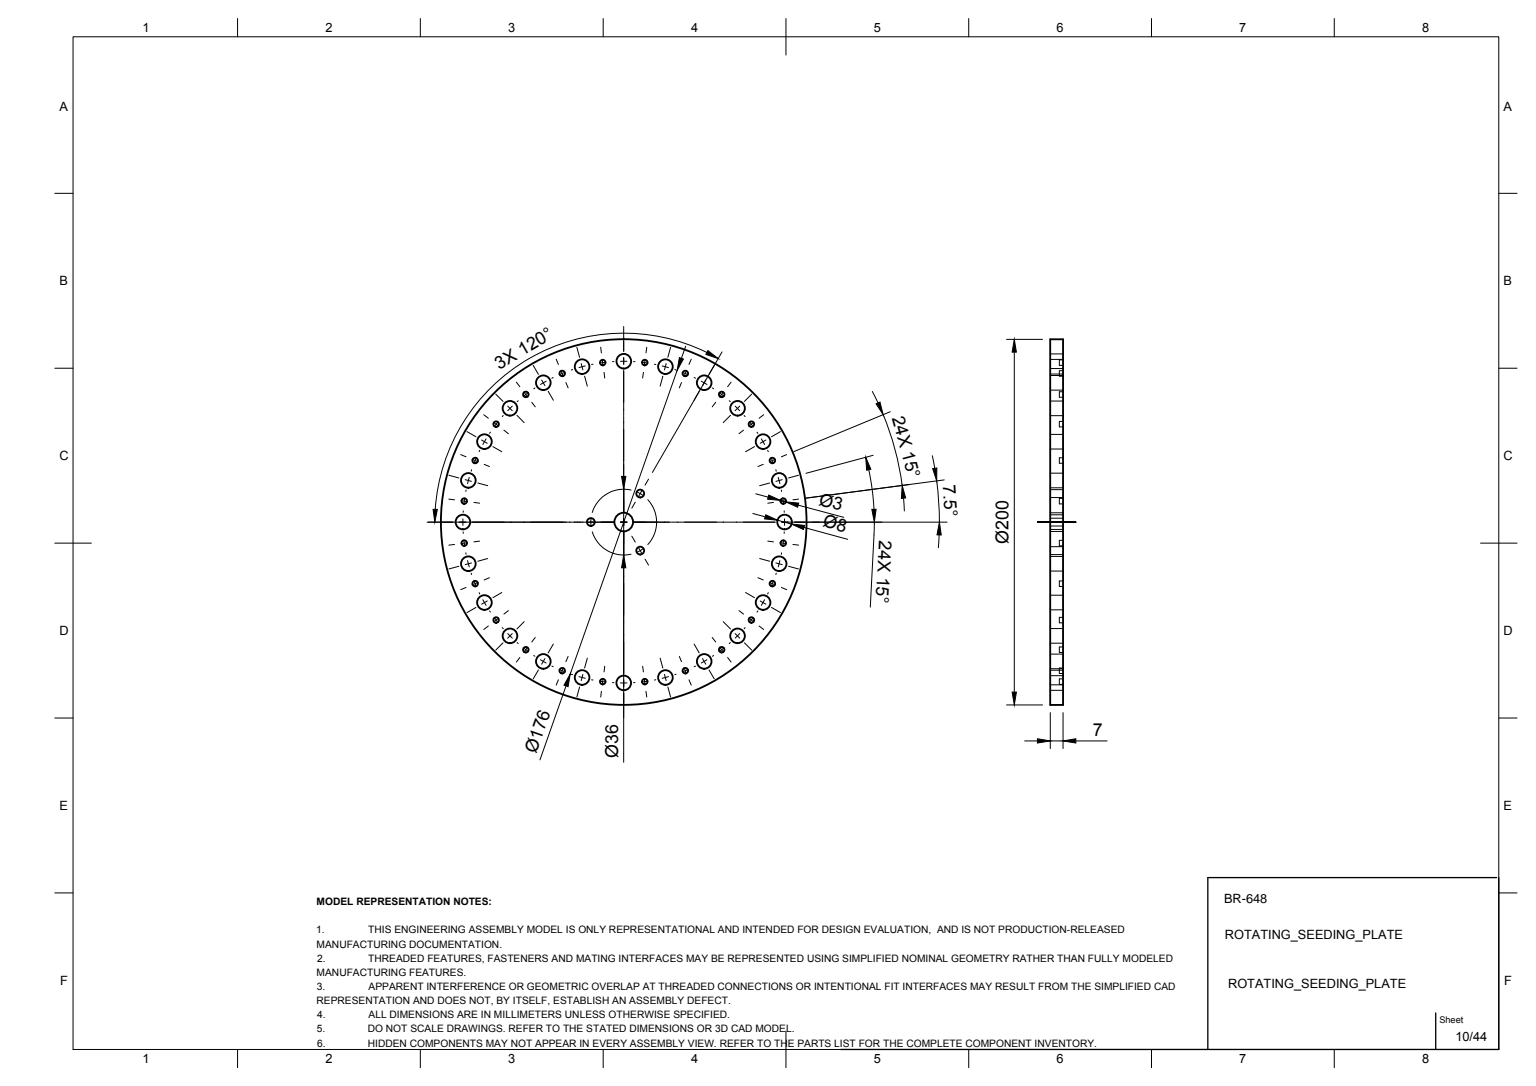
ISO-10303-21;
HEADER;
FILE_DESCRIPTION((''),'2;1');
FILE_NAME('ROTATING_SEEDING_PLATE.step','2026-10-01T22:05:39-07:00',(''),(''),'','','');
FILE_SCHEMA (('AUTOMOTIVE_DESIGN { 1 0 10303 214 3 1 1 }'));
ENDSEC;
DATA;
#10=MECHANICAL_DESIGN_GEOMETRIC_PRESENTATION_REPRESENTATION('',(#610),#24628);
#526=SHAPE_REPRESENTATION_RELATIONSHIP('SRR','None',#24798,#568) ;
#568=ADVANCED_BREP_SHAPE_REPRESENTATION('',(#652),#24588) ;
#610=STYLED_ITEM('',(#25034),#652) ;
#652=MANIFOLD_SOLID_BREP('ROTATING_SEEDING_PLATE',#13119) ;
#759=FACE_BOUND('',#3963,.T.) ;
#760=FACE_BOUND('',#3964,.T.) ;
#761=FACE_BOUND('',#3965,.T.) ;
#762=FACE_BOUND('',#3966,.T.) ;
#763=FACE_BOUND('',#3967,.T.) ;
#764=FACE_BOUND('',#3968,.T.) ;
#765=FACE_BOUND('',#3969,.T.) ;
#766=FACE_BOUND('',#3970,.T.) ;
#767=FACE_BOUND('',#3971,.T.) ;
#768=FACE_BOUND('',#3972,.T.) ;
#769=FACE_BOUND('',#3973,.T.) ;
#770=FACE_BOUND('',#3974,.T.) ;
#771=FACE_BOUND('',#3975,.T.) ;
#772=FACE_BOUND('',#3976,.T.) ;
#773=FACE_BOUND('',#3977,.T.) ;
#774=FACE_BOUND('',#3978,.T.) ;
#775=FACE_BOUND('',#3979,.T.) ;
#776=FACE_BOUND('',#3980,.T.) ;
#777=FACE_BOUND('',#3981,.T.) ;
#778=FACE_BOUND('',#3982,.T.) ;
#779=FACE_BOUND('',#3983,.T.) ;
#780=FACE_BOUND('',#3984,.T.) ;
#781=FACE_BOUND('',#3985,.T.) ;
#782=FACE_BOUND('',#3986,.T.) ;
#783=FACE_BOUND('',#3987,.T.) ;
#784=FACE_BOUND('',#3988,.T.) ;
#785=FACE_BOUND('',#3989,.T.) ;
#786=FACE_BOUND('',#3990,.T.) ;
#787=FACE_BOUND('',#3991,.T.) ;
#788=FACE_BOUND('',#3992,.T.) ;
#789=FACE_BOUND('',#3993,.T.) ;
#790=FACE_BOUND('',#3994,.T.) ;
#791=FACE_BOUND('',#3995,.T.) ;
#792=FACE_BOUND('',#3996,.T.) ;
#793=FACE_BOUND('',#3997,.T.) ;
#794=FACE_BOUND('',#3998,.T.) ;
#795=FACE_BOUND('',#3999,.T.) ;
#796=FACE_BOUND('',#4000,.T.) ;
#797=FACE_BOUND('',#4001,.T.) ;
#798=FACE_BOUND('',#4002,.T.) ;
#799=FACE_BOUND('',#4003,.T.) ;
#800=FACE_BOUND('',#4004,.T.) ;
#801=FACE_BOUND('',#4005,.T.) ;
#802=FACE_BOUND('',#4006,.T.) ;
#803=FACE_BOUND('',#4007,.T.) ;
#804=FACE_BOUND('',#4008,.T.) ;
#805=FACE_BOUND('',#4009,.T.) ;
#806=FACE_BOUND('',#4010,.T.) ;
#807=FACE_BOUND('',#4011,.T.) ;
#808=FACE_BOUND('',#4012,.T.) ;
#809=FACE_BOUND('',#4013,.T.) ;
#810=FACE_BOUND('',#4014,.T.) ;
#811=FACE_BOUND('',#4016,.T.) ;
#812=FACE_BOUND('',#4017,.T.) ;
#813=FACE_BOUND('',#4018,.T.) ;
#814=FACE_BOUND('',#4019,.T.) ;
#815=FACE_BOUND('',#4020,.T.) ;
#816=FACE_BOUND('',#4021,.T.) ;
#817=FACE_BOUND('',#4022,.T.) ;
#818=FACE_BOUND('',#4023,.T.) ;
#819=FACE_BOUND('',#4024,.T.) ;
#820=FACE_BOUND('',#4025,.T.) ;
#821=FACE_BOUND('',#4026,.T.) ;
#822=FACE_BOUND('',#4027,.T.) ;
#823=FACE_BOUND('',#4028,.T.) ;
#824=FACE_BOUND('',#4029,.T.) ;
#825=FACE_BOUND('',#4030,.T.) ;
#826=FACE_BOUND('',#4031,.T.) ;
#827=FACE_BOUND('',#4032,.T.) ;
#828=FACE_BOUND('',#4033,.T.) ;
#829=FACE_BOUND('',#4034,.T.) ;
#830=FACE_BOUND('',#4035,.T.) ;
#831=FACE_BOUND('',#4036,.T.) ;
#832=FACE_BOUND('',#4037,.T.) ;
#833=FACE_BOUND('',#4038,.T.) ;
#834=FACE_BOUND('',#4039,.T.) ;
#835=FACE_BOUND('',#4040,.T.) ;
#836=FACE_BOUND('',#4041,.T.) ;
#837=FACE_BOUND('',#4042,.T.) ;
#838=FACE_BOUND('',#4043,.T.) ;
#1089=LINE('',#20269,#1925) ;
#1090=LINE('',#20276,#1926) ;
#1091=LINE('',#20283,#1927) ;
#1092=LINE('',#20290,#1928) ;
#1093=LINE('',#20297,#1929) ;
#1094=LINE('',#20304,#1930) ;
#1095=LINE('',#20311,#1931) ;
#1096=LINE('',#20318,#1932) ;
#1097=LINE('',#20325,#1933) ;
#1098=LINE('',#20332,#1934) ;
#1099=LINE('',#20339,#1935) ;
#1100=LINE('',#20346,#1936) ;
#1101=LINE('',#20353,#1937) ;
#1102=LINE('',#20360,#1938) ;
#1103=LINE('',#20367,#1939) ;
#1104=LINE('',#20374,#1940) ;
#1105=LINE('',#20381,#1941) ;
#1106=LINE('',#20388,#1942) ;
#1107=LINE('',#20395,#1943) ;
#1108=LINE('',#20402,#1944) ;
#1109=LINE('',#20409,#1945) ;
#1110=LINE('',#20416,#1946) ;
#1111=LINE('',#20423,#1947) ;
#1112=LINE('',#20430,#1948) ;
#1113=LINE('',#20437,#1949) ;
#1114=LINE('',#20443,#1950) ;
#1115=LINE('',#20449,#1951) ;
#1116=LINE('',#20455,#1952) ;
#1117=LINE('',#20461,#1953) ;
#1118=LINE('',#20467,#1954) ;
#1119=LINE('',#20473,#1955) ;
#1120=LINE('',#20479,#1956) ;
#1121=LINE('',#20485,#1957) ;
#1122=LINE('',#20491,#1958) ;
#1123=LINE('',#20497,#1959) ;
#1124=LINE('',#20503,#1960) ;
#1125=LINE('',#20509,#1961) ;
#1126=LINE('',#20515,#1962) ;
#1127=LINE('',#20521,#1963) ;
#1128=LINE('',#20527,#1964) ;
#1129=LINE('',#20533,#1965) ;
#1130=LINE('',#20539,#1966) ;
#1131=LINE('',#20545,#1967) ;
#1132=LINE('',#20551,#1968) ;
#1133=LINE('',#20557,#1969) ;
#1134=LINE('',#20563,#1970) ;
#1135=LINE('',#20569,#1971) ;
#1136=LINE('',#20575,#1972) ;
#1137=LINE('',#20581,#1973) ;
#1138=LINE('',#20587,#1974) ;
#1139=LINE('',#20593,#1975) ;
#1140=LINE('',#20599,#1976) ;
#1141=LINE('',#20605,#1977) ;
#1925=VECTOR('',#15930,0.15) ;
#1926=VECTOR('',#15939,0.15) ;
#1927=VECTOR('',#15948,0.15) ;
#1928=VECTOR('',#15957,0.15) ;
#1929=VECTOR('',#15966,0.15) ;
#1930=VECTOR('',#15975,0.15) ;
#1931=VECTOR('',#15984,0.15) ;
#1932=VECTOR('',#15993,0.15) ;
#1933=VECTOR('',#16002,0.15) ;
#1934=VECTOR('',#16011,0.15) ;
#1935=VECTOR('',#16020,0.15) ;
#1936=VECTOR('',#16029,0.15) ;
#1937=VECTOR('',#16038,0.15) ;
#1938=VECTOR('',#16047,0.15) ;
#1939=VECTOR('',#16056,0.15) ;
#1940=VECTOR('',#16065,0.15) ;
#1941=VECTOR('',#16074,0.15) ;
#1942=VECTOR('',#16083,0.15) ;
#1943=VECTOR('',#16092,0.15) ;
#1944=VECTOR('',#16101,0.15) ;
#1945=VECTOR('',#16110,0.15) ;
#1946=VECTOR('',#16119,0.15) ;
#1947=VECTOR('',#16128,0.15) ;
#1948=VECTOR('',#16137,0.15) ;
#1949=VECTOR('',#16146,0.4) ;
#1950=VECTOR('',#16153,0.4) ;
#1951=VECTOR('',#16160,0.4) ;
#1952=VECTOR('',#16167,0.4) ;
#1953=VECTOR('',#16174,0.4) ;
#1954=VECTOR('',#16181,0.4) ;
#1955=VECTOR('',#16188,0.4) ;
#1956=VECTOR('',#16195,0.4) ;
#1957=VECTOR('',#16202,0.4) ;
#1958=VECTOR('',#16209,0.4) ;
#1959=VECTOR('',#16216,0.4) ;
#1960=VECTOR('',#16223,0.4) ;
#1961=VECTOR('',#16230,0.4) ;
#1962=VECTOR('',#16237,0.4) ;
#1963=VECTOR('',#16244,0.4) ;
#1964=VECTOR('',#16251,0.4) ;
#1965=VECTOR('',#16258,0.4) ;
#1966=VECTOR('',#16265,0.4) ;
#1967=VECTOR('',#16272,0.4) ;
#1968=VECTOR('',#16279,0.4) ;
#1969=VECTOR('',#16286,0.4) ;
#1970=VECTOR('',#16293,0.4) ;
#1971=VECTOR('',#16300,0.4) ;
#1972=VECTOR('',#16307,0.4) ;
#1973=VECTOR('',#16314,0.215) ;
#1974=VECTOR('',#16321,0.215) ;
#1975=VECTOR('',#16328,0.215) ;
#1976=VECTOR('',#16335,0.51) ;
#1977=VECTOR('',#16342,10.) ;
#2725=CYLINDRICAL_SURFACE('',#13876,0.15) ;
#2726=CYLINDRICAL_SURFACE('',#13880,0.15) ;
#2727=CYLINDRICAL_SURFACE('',#13884,0.15) ;
#2728=CYLINDRICAL_SURFACE('',#13888,0.15) ;
#2729=CYLINDRICAL_SURFACE('',#13892,0.15) ;
#2730=CYLINDRICAL_SURFACE('',#13896,0.15) ;
#2731=CYLINDRICAL_SURFACE('',#13900,0.15) ;
#2732=CYLINDRICAL_SURFACE('',#13904,0.15) ;
#2733=CYLINDRICAL_SURFACE('',#13908,0.15) ;
#2734=CYLINDRICAL_SURFACE('',#13912,0.15) ;
#2735=CYLINDRICAL_SURFACE('',#13916,0.15) ;
#2736=CYLINDRICAL_SURFACE('',#13920,0.15) ;
#2737=CYLINDRICAL_SURFACE('',#13924,0.15) ;
#2738=CYLINDRICAL_SURFACE('',#13928,0.15) ;
#2739=CYLINDRICAL_SURFACE('',#13932,0.15) ;
#2740=CYLINDRICAL_SURFACE('',#13936,0.15) ;
#2741=CYLINDRICAL_SURFACE('',#13940,0.15) ;
#2742=CYLINDRICAL_SURFACE('',#13944,0.15) ;
#2743=CYLINDRICAL_SURFACE('',#13948,0.15) ;
#2744=CYLINDRICAL_SURFACE('',#13952,0.15) ;
#2745=CYLINDRICAL_SURFACE('',#13956,0.15) ;
#2746=CYLINDRICAL_SURFACE('',#13960,0.15) ;
#2747=CYLINDRICAL_SURFACE('',#13964,0.15) ;
#2748=CYLINDRICAL_SURFACE('',#13968,0.15) ;
#2749=CYLINDRICAL_SURFACE('',#13972,0.4) ;
#2750=CYLINDRICAL_SURFACE('',#13975,0.4) ;
#2751=CYLINDRICAL_SURFACE('',#13978,0.4) ;
#2752=CYLINDRICAL_SURFACE('',#13981,0.4) ;
#2753=CYLINDRICAL_SURFACE('',#13984,0.4) ;
#2754=CYLINDRICAL_SURFACE('',#13987,0.4) ;
#2755=CYLINDRICAL_SURFACE('',#13990,0.4) ;
#2756=CYLINDRICAL_SURFACE('',#13993,0.4) ;
#2757=CYLINDRICAL_SURFACE('',#13996,0.4) ;
#2758=CYLINDRICAL_SURFACE('',#13999,0.4) ;
#2759=CYLINDRICAL_SURFACE('',#14002,0.4) ;
#2760=CYLINDRICAL_SURFACE('',#14005,0.4) ;
#2761=CYLINDRICAL_SURFACE('',#14008,0.4) ;
#2762=CYLINDRICAL_SURFACE('',#14011,0.4) ;
#2763=CYLINDRICAL_SURFACE('',#14014,0.4) ;
#2764=CYLINDRICAL_SURFACE('',#14017,0.4) ;
#2765=CYLINDRICAL_SURFACE('',#14020,0.4) ;
#2766=CYLINDRICAL_SURFACE('',#14023,0.4) ;
#2767=CYLINDRICAL_SURFACE('',#14026,0.4) ;
#2768=CYLINDRICAL_SURFACE('',#14029,0.4) ;
#2769=CYLINDRICAL_SURFACE('',#14032,0.4) ;
#2770=CYLINDRICAL_SURFACE('',#14035,0.4) ;
#2771=CYLINDRICAL_SURFACE('',#14038,0.4) ;
#2772=CYLINDRICAL_SURFACE('',#14041,0.4) ;
#2773=CYLINDRICAL_SURFACE('',#14044,0.215) ;
#2774=CYLINDRICAL_SURFACE('',#14047,0.215) ;
#2775=CYLINDRICAL_SURFACE('',#14050,0.215) ;
#2776=CYLINDRICAL_SURFACE('',#14053,0.51) ;
#2777=CYLINDRICAL_SURFACE('',#14056,10.) ;
#3045=FACE_OUTER_BOUND('',#3885,.T.) ;
#3046=FACE_OUTER_BOUND('',#3886,.T.) ;
#3047=FACE_OUTER_BOUND('',#3887,.T.) ;
#3048=FACE_OUTER_BOUND('',#3888,.T.) ;
#3049=FACE_OUTER_BOUND('',#3889,.T.) ;
#3050=FACE_OUTER_BOUND('',#3890,.T.) ;
#3051=FACE_OUTER_BOUND('',#3891,.T.) ;
#3052=FACE_OUTER_BOUND('',#3892,.T.) ;
#3053=FACE_OUTER_BOUND('',#3893,.T.) ;
#3054=FACE_OUTER_BOUND('',#3894,.T.) ;
#3055=FACE_OUTER_BOUND('',#3895,.T.) ;
#3056=FACE_OUTER_BOUND('',#3896,.T.) ;
#3057=FACE_OUTER_BOUND('',#3897,.T.) ;
#3058=FACE_OUTER_BOUND('',#3898,.T.) ;
#3059=FACE_OUTER_BOUND('',#3899,.T.) ;
#3060=FACE_OUTER_BOUND('',#3900,.T.) ;
#3061=FACE_OUTER_BOUND('',#3901,.T.) ;
#3062=FACE_OUTER_BOUND('',#3902,.T.) ;
#3063=FACE_OUTER_BOUND('',#3903,.T.) ;
#3064=FACE_OUTER_BOUND('',#3904,.T.) ;
#3065=FACE_OUTER_BOUND('',#3905,.T.) ;
#3066=FACE_OUTER_BOUND('',#3906,.T.) ;
#3067=FACE_OUTER_BOUND('',#3907,.T.) ;
#3068=FACE_OUTER_BOUND('',#3908,.T.) ;
#3069=FACE_OUTER_BOUND('',#3909,.T.) ;
#3070=FACE_OUTER_BOUND('',#3910,.T.) ;
#3071=FACE_OUTER_BOUND('',#3911,.T.) ;
#3072=FACE_OUTER_BOUND('',#3912,.T.) ;
#3073=FACE_OUTER_BOUND('',#3913,.T.) ;
#3074=FACE_OUTER_BOUND('',#3914,.T.) ;
#3075=FACE_OUTER_BOUND('',#3915,.T.) ;
#3076=FACE_OUTER_BOUND('',#3916,.T.) ;
#3077=FACE_OUTER_BOUND('',#3917,.T.) ;
#3078=FACE_OUTER_BOUND('',#3918,.T.) ;
#3079=FACE_OUTER_BOUND('',#3919,.T.) ;
#3080=FACE_OUTER_BOUND('',#3920,.T.) ;
#3081=FACE_OUTER_BOUND('',#3921,.T.) ;
#3082=FACE_OUTER_BOUND('',#3922,.T.) ;
#3083=FACE_OUTER_BOUND('',#3923,.T.) ;
#3084=FACE_OUTER_BOUND('',#3924,.T.) ;
#3085=FACE_OUTER_BOUND('',#3925,.T.) ;
#3086=FACE_OUTER_BOUND('',#3926,.T.) ;
#3087=FACE_OUTER_BOUND('',#3927,.T.) ;
#3088=FACE_OUTER_BOUND('',#3928,.T.) ;
#3089=FACE_OUTER_BOUND('',#3929,.T.) ;
#3090=FACE_OUTER_BOUND('',#3930,.T.) ;
#3091=FACE_OUTER_BOUND('',#3931,.T.) ;
#3092=FACE_OUTER_BOUND('',#3932,.T.) ;
#3093=FACE_OUTER_BOUND('',#3933,.T.) ;
#3094=FACE_OUTER_BOUND('',#3934,.T.) ;
#3095=FACE_OUTER_BOUND('',#3935,.T.) ;
#3096=FACE_OUTER_BOUND('',#3936,.T.) ;
#3097=FACE_OUTER_BOUND('',#3937,.T.) ;
#3098=FACE_OUTER_BOUND('',#3938,.T.) ;
#3099=FACE_OUTER_BOUND('',#3939,.T.) ;
#3100=FACE_OUTER_BOUND('',#3940,.T.) ;
#3101=FACE_OUTER_BOUND('',#3941,.T.) ;
#3102=FACE_OUTER_BOUND('',#3942,.T.) ;
#3103=FACE_OUTER_BOUND('',#3943,.T.) ;
#3104=FACE_OUTER_BOUND('',#3944,.T.) ;
#3105=FACE_OUTER_BOUND('',#3945,.T.) ;
#3106=FACE_OUTER_BOUND('',#3946,.T.) ;
#3107=FACE_OUTER_BOUND('',#3947,.T.) ;
#3108=FACE_OUTER_BOUND('',#3948,.T.) ;
#3109=FACE_OUTER_BOUND('',#3949,.T.) ;
#3110=FACE_OUTER_BOUND('',#3950,.T.) ;
#3111=FACE_OUTER_BOUND('',#3951,.T.) ;
#3112=FACE_OUTER_BOUND('',#3952,.T.) ;
#3113=FACE_OUTER_BOUND('',#3953,.T.) ;
#3114=FACE_OUTER_BOUND('',#3954,.T.) ;
#3115=FACE_OUTER_BOUND('',#3955,.T.) ;
#3116=FACE_OUTER_BOUND('',#3956,.T.) ;
#3117=FACE_OUTER_BOUND('',#3957,.T.) ;
#3118=FACE_OUTER_BOUND('',#3958,.T.) ;
#3119=FACE_OUTER_BOUND('',#3959,.T.) ;
#3120=FACE_OUTER_BOUND('',#3960,.T.) ;
#3121=FACE_OUTER_BOUND('',#3961,.T.) ;
#3122=FACE_OUTER_BOUND('',#3962,.T.) ;
#3123=FACE_OUTER_BOUND('',#4015,.T.) ;
#3885=EDGE_LOOP('',(#8919,#8920,#8921,#8922)) ;
#3886=EDGE_LOOP('',(#8923)) ;
#3887=EDGE_LOOP('',(#8924,#8925,#8926,#8927)) ;
#3888=EDGE_LOOP('',(#8928)) ;
#3889=EDGE_LOOP('',(#8929,#8930,#8931,#8932)) ;
#3890=EDGE_LOOP('',(#8933)) ;
#3891=EDGE_LOOP('',(#8934,#8935,#8936,#8937)) ;
#3892=EDGE_LOOP('',(#8938)) ;
#3893=EDGE_LOOP('',(#8939,#8940,#8941,#8942)) ;
#3894=EDGE_LOOP('',(#8943)) ;
#3895=EDGE_LOOP('',(#8944,#8945,#8946,#8947)) ;
#3896=EDGE_LOOP('',(#8948)) ;
#3897=EDGE_LOOP('',(#8949,#8950,#8951,#8952)) ;
#3898=EDGE_LOOP('',(#8953)) ;
#3899=EDGE_LOOP('',(#8954,#8955,#8956,#8957)) ;
#3900=EDGE_LOOP('',(#8958)) ;
#3901=EDGE_LOOP('',(#8959,#8960,#8961,#8962)) ;
#3902=EDGE_LOOP('',(#8963)) ;
#3903=EDGE_LOOP('',(#8964,#8965,#8966,#8967)) ;
#3904=EDGE_LOOP('',(#8968)) ;
#3905=EDGE_LOOP('',(#8969,#8970,#8971,#8972)) ;
#3906=EDGE_LOOP('',(#8973)) ;
#3907=EDGE_LOOP('',(#8974,#8975,#8976,#8977)) ;
#3908=EDGE_LOOP('',(#8978)) ;
#3909=EDGE_LOOP('',(#8979,#8980,#8981,#8982)) ;
#3910=EDGE_LOOP('',(#8983)) ;
#3911=EDGE_LOOP('',(#8984,#8985,#8986,#8987)) ;
#3912=EDGE_LOOP('',(#8988)) ;
#3913=EDGE_LOOP('',(#8989,#8990,#8991,#8992)) ;
#3914=EDGE_LOOP('',(#8993)) ;
#3915=EDGE_LOOP('',(#8994,#8995,#8996,#8997)) ;
#3916=EDGE_LOOP('',(#8998)) ;
#3917=EDGE_LOOP('',(#8999,#9000,#9001,#9002)) ;
#3918=EDGE_LOOP('',(#9003)) ;
#3919=EDGE_LOOP('',(#9004,#9005,#9006,#9007)) ;
#3920=EDGE_LOOP('',(#9008)) ;
#3921=EDGE_LOOP('',(#9009,#9010,#9011,#9012)) ;
#3922=EDGE_LOOP('',(#9013)) ;
#3923=EDGE_LOOP('',(#9014,#9015,#9016,#9017)) ;
#3924=EDGE_LOOP('',(#9018)) ;
#3925=EDGE_LOOP('',(#9019,#9020,#9021,#9022)) ;
#3926=EDGE_LOOP('',(#9023)) ;
#3927=EDGE_LOOP('',(#9024,#9025,#9026,#9027)) ;
#3928=EDGE_LOOP('',(#9028)) ;
#3929=EDGE_LOOP('',(#9029,#9030,#9031,#9032)) ;
#3930=EDGE_LOOP('',(#9033)) ;
#3931=EDGE_LOOP('',(#9034,#9035,#9036,#9037)) ;
#3932=EDGE_LOOP('',(#9038)) ;
#3933=EDGE_LOOP('',(#9039,#9040,#9041,#9042)) ;
#3934=EDGE_LOOP('',(#9043,#9044,#9045,#9046)) ;
#3935=EDGE_LOOP('',(#9047,#9048,#9049,#9050)) ;
#3936=EDGE_LOOP('',(#9051,#9052,#9053,#9054)) ;
#3937=EDGE_LOOP('',(#9055,#9056,#9057,#9058)) ;
#3938=EDGE_LOOP('',(#9059,#9060,#9061,#9062)) ;
#3939=EDGE_LOOP('',(#9063,#9064,#9065,#9066)) ;
#3940=EDGE_LOOP('',(#9067,#9068,#9069,#9070)) ;
#3941=EDGE_LOOP('',(#9071,#9072,#9073,#9074)) ;
#3942=EDGE_LOOP('',(#9075,#9076,#9077,#9078)) ;
#3943=EDGE_LOOP('',(#9079,#9080,#9081,#9082)) ;
#3944=EDGE_LOOP('',(#9083,#9084,#9085,#9086)) ;
#3945=EDGE_LOOP('',(#9087,#9088,#9089,#9090)) ;
#3946=EDGE_LOOP('',(#9091,#9092,#9093,#9094)) ;
#3947=EDGE_LOOP('',(#9095,#9096,#9097,#9098)) ;
#3948=EDGE_LOOP('',(#9099,#9100,#9101,#9102)) ;
#3949=EDGE_LOOP('',(#9103,#9104,#9105,#9106)) ;
#3950=EDGE_LOOP('',(#9107,#9108,#9109,#9110)) ;
#3951=EDGE_LOOP('',(#9111,#9112,#9113,#9114)) ;
#3952=EDGE_LOOP('',(#9115,#9116,#9117,#9118)) ;
#3953=EDGE_LOOP('',(#9119,#9120,#9121,#9122)) ;
#3954=EDGE_LOOP('',(#9123,#9124,#9125,#9126)) ;
#3955=EDGE_LOOP('',(#9127,#9128,#9129,#9130)) ;
#3956=EDGE_LOOP('',(#9131,#9132,#9133,#9134)) ;
#3957=EDGE_LOOP('',(#9135,#9136,#9137,#9138)) ;
#3958=EDGE_LOOP('',(#9139,#9140,#9141,#9142)) ;
#3959=EDGE_LOOP('',(#9143,#9144,#9145,#9146)) ;
#3960=EDGE_LOOP('',(#9147,#9148,#9149,#9150)) ;
#3961=EDGE_LOOP('',(#9151,#9152,#9153,#9154)) ;
#3962=EDGE_LOOP('',(#9155)) ;
#3963=EDGE_LOOP('',(#9156)) ;
#3964=EDGE_LOOP('',(#9157)) ;
#3965=EDGE_LOOP('',(#9158)) ;
#3966=EDGE_LOOP('',(#9159)) ;
#3967=EDGE_LOOP('',(#9160)) ;
#3968=EDGE_LOOP('',(#9161)) ;
#3969=EDGE_LOOP('',(#9162)) ;
#3970=EDGE_LOOP('',(#9163)) ;
#3971=EDGE_LOOP('',(#9164)) ;
#3972=EDGE_LOOP('',(#9165)) ;
#3973=EDGE_LOOP('',(#9166)) ;
#3974=EDGE_LOOP('',(#9167)) ;
#3975=EDGE_LOOP('',(#9168)) ;
#3976=EDGE_LOOP('',(#9169)) ;
#3977=EDGE_LOOP('',(#9170)) ;
#3978=EDGE_LOOP('',(#9171)) ;
#3979=EDGE_LOOP('',(#9172)) ;
#3980=EDGE_LOOP('',(#9173)) ;
#3981=EDGE_LOOP('',(#9174)) ;
#3982=EDGE_LOOP('',(#9175)) ;
#3983=EDGE_LOOP('',(#9176)) ;
#3984=EDGE_LOOP('',(#9177)) ;
#3985=EDGE_LOOP('',(#9178)) ;
#3986=EDGE_LOOP('',(#9179)) ;
#3987=EDGE_LOOP('',(#9180)) ;
#3988=EDGE_LOOP('',(#9181)) ;
#3989=EDGE_LOOP('',(#9182)) ;
#3990=EDGE_LOOP('',(#9183)) ;
#3991=EDGE_LOOP('',(#9184)) ;
#3992=EDGE_LOOP('',(#9185)) ;
#3993=EDGE_LOOP('',(#9186)) ;
#3994=EDGE_LOOP('',(#9187)) ;
#3995=EDGE_LOOP('',(#9188)) ;
#3996=EDGE_LOOP('',(#9189)) ;
#3997=EDGE_LOOP('',(#9190)) ;
#3998=EDGE_LOOP('',(#9191)) ;
#3999=EDGE_LOOP('',(#9192)) ;
#4000=EDGE_LOOP('',(#9193)) ;
#4001=EDGE_LOOP('',(#9194)) ;
#4002=EDGE_LOOP('',(#9195)) ;
#4003=EDGE_LOOP('',(#9196)) ;
#4004=EDGE_LOOP('',(#9197)) ;
#4005=EDGE_LOOP('',(#9198)) ;
#4006=EDGE_LOOP('',(#9199)) ;
#4007=EDGE_LOOP('',(#9200)) ;
#4008=EDGE_LOOP('',(#9201)) ;
#4009=EDGE_LOOP('',(#9202)) ;
#4010=EDGE_LOOP('',(#9203)) ;
#4011=EDGE_LOOP('',(#9204)) ;
#4012=EDGE_LOOP('',(#9205)) ;
#4013=EDGE_LOOP('',(#9206)) ;
#4014=EDGE_LOOP('',(#9207)) ;
#4015=EDGE_LOOP('',(#9208)) ;
#4016=EDGE_LOOP('',(#9209)) ;
#4017=EDGE_LOOP('',(#9210)) ;
#4018=EDGE_LOOP('',(#9211)) ;
#4019=EDGE_LOOP('',(#9212)) ;
#4020=EDGE_LOOP('',(#9213)) ;
#4021=EDGE_LOOP('',(#9214)) ;
#4022=EDGE_LOOP('',(#9215)) ;
#4023=EDGE_LOOP('',(#9216)) ;
#4024=EDGE_LOOP('',(#9217)) ;
#4025=EDGE_LOOP('',(#9218)) ;
#4026=EDGE_LOOP('',(#9219)) ;
#4027=EDGE_LOOP('',(#9220)) ;
#4028=EDGE_LOOP('',(#9221)) ;
#4029=EDGE_LOOP('',(#9222)) ;
#4030=EDGE_LOOP('',(#9223)) ;
#4031=EDGE_LOOP('',(#9224)) ;
#4032=EDGE_LOOP('',(#9225)) ;
#4033=EDGE_LOOP('',(#9226)) ;
#4034=EDGE_LOOP('',(#9227)) ;
#4035=EDGE_LOOP('',(#9228)) ;
#4036=EDGE_LOOP('',(#9229)) ;
#4037=EDGE_LOOP('',(#9230)) ;
#4038=EDGE_LOOP('',(#9231)) ;
#4039=EDGE_LOOP('',(#9232)) ;
#4040=EDGE_LOOP('',(#9233)) ;
#4041=EDGE_LOOP('',(#9234)) ;
#4042=EDGE_LOOP('',(#9235)) ;
#4043=EDGE_LOOP('',(#9236)) ;
#4874=CIRCLE('',#13877,0.15) ;
#4875=CIRCLE('',#13878,0.15) ;
#4876=CIRCLE('',#13881,0.15) ;
#4877=CIRCLE('',#13882,0.15) ;
#4878=CIRCLE('',#13885,0.15) ;
#4879=CIRCLE('',#13886,0.15) ;
#4880=CIRCLE('',#13889,0.15) ;
#4881=CIRCLE('',#13890,0.15) ;
#4882=CIRCLE('',#13893,0.15) ;
#4883=CIRCLE('',#13894,0.15) ;
#4884=CIRCLE('',#13897,0.15) ;
#4885=CIRCLE('',#13898,0.15) ;
#4886=CIRCLE('',#13901,0.15) ;
#4887=CIRCLE('',#13902,0.15) ;
#4888=CIRCLE('',#13905,0.15) ;
#4889=CIRCLE('',#13906,0.15) ;
#4890=CIRCLE('',#13909,0.15) ;
#4891=CIRCLE('',#13910,0.15) ;
#4892=CIRCLE('',#13913,0.15) ;
#4893=CIRCLE('',#13914,0.15) ;
#4894=CIRCLE('',#13917,0.15) ;
#4895=CIRCLE('',#13918,0.15) ;
#4896=CIRCLE('',#13921,0.15) ;
#4897=CIRCLE('',#13922,0.15) ;
#4898=CIRCLE('',#13925,0.15) ;
#4899=CIRCLE('',#13926,0.15) ;
#4900=CIRCLE('',#13929,0.15) ;
#4901=CIRCLE('',#13930,0.15) ;
#4902=CIRCLE('',#13933,0.15) ;
#4903=CIRCLE('',#13934,0.15) ;
#4904=CIRCLE('',#13937,0.15) ;
#4905=CIRCLE('',#13938,0.15) ;
#4906=CIRCLE('',#13941,0.15) ;
#4907=CIRCLE('',#13942,0.15) ;
#4908=CIRCLE('',#13945,0.15) ;
#4909=CIRCLE('',#13946,0.15) ;
#4910=CIRCLE('',#13949,0.15) ;
#4911=CIRCLE('',#13950,0.15) ;
#4912=CIRCLE('',#13953,0.15) ;
#4913=CIRCLE('',#13954,0.15) ;
#4914=CIRCLE('',#13957,0.15) ;
#4915=CIRCLE('',#13958,0.15) ;
#4916=CIRCLE('',#13961,0.15) ;
#4917=CIRCLE('',#13962,0.15) ;
#4918=CIRCLE('',#13965,0.15) ;
#4919=CIRCLE('',#13966,0.15) ;
#4920=CIRCLE('',#13969,0.15) ;
#4921=CIRCLE('',#13970,0.15) ;
#4922=CIRCLE('',#13973,0.4) ;
#4923=CIRCLE('',#13974,0.4) ;
#4924=CIRCLE('',#13976,0.4) ;
#4925=CIRCLE('',#13977,0.4) ;
#4926=CIRCLE('',#13979,0.4) ;
#4927=CIRCLE('',#13980,0.4) ;
#4928=CIRCLE('',#13982,0.4) ;
#4929=CIRCLE('',#13983,0.4) ;
#4930=CIRCLE('',#13985,0.4) ;
#4931=CIRCLE('',#13986,0.4) ;
#4932=CIRCLE('',#13988,0.4) ;
#4933=CIRCLE('',#13989,0.4) ;
#4934=CIRCLE('',#13991,0.4) ;
#4935=CIRCLE('',#13992,0.4) ;
#4936=CIRCLE('',#13994,0.4) ;
#4937=CIRCLE('',#13995,0.4) ;
#4938=CIRCLE('',#13997,0.4) ;
#4939=CIRCLE('',#13998,0.4) ;
#4940=CIRCLE('',#14000,0.4) ;
#4941=CIRCLE('',#14001,0.4) ;
#4942=CIRCLE('',#14003,0.4) ;
#4943=CIRCLE('',#14004,0.4) ;
#4944=CIRCLE('',#14006,0.4) ;
#4945=CIRCLE('',#14007,0.4) ;
#4946=CIRCLE('',#14009,0.4) ;
#4947=CIRCLE('',#14010,0.4) ;
#4948=CIRCLE('',#14012,0.4) ;
#4949=CIRCLE('',#14013,0.4) ;
#4950=CIRCLE('',#14015,0.4) ;
#4951=CIRCLE('',#14016,0.4) ;
#4952=CIRCLE('',#14018,0.4) ;
#4953=CIRCLE('',#14019,0.4) ;
#4954=CIRCLE('',#14021,0.4) ;
#4955=CIRCLE('',#14022,0.4) ;
#4956=CIRCLE('',#14024,0.4) ;
#4957=CIRCLE('',#14025,0.4) ;
#4958=CIRCLE('',#14027,0.4) ;
#4959=CIRCLE('',#14028,0.4) ;
#4960=CIRCLE('',#14030,0.4) ;
#4961=CIRCLE('',#14031,0.4) ;
#4962=CIRCLE('',#14033,0.4) ;
#4963=CIRCLE('',#14034,0.4) ;
#4964=CIRCLE('',#14036,0.4) ;
#4965=CIRCLE('',#14037,0.4) ;
#4966=CIRCLE('',#14039,0.4) ;
#4967=CIRCLE('',#14040,0.4) ;
#4968=CIRCLE('',#14042,0.4) ;
#4969=CIRCLE('',#14043,0.4) ;
#4970=CIRCLE('',#14045,0.215) ;
#4971=CIRCLE('',#14046,0.215) ;
#4972=CIRCLE('',#14048,0.215) ;
#4973=CIRCLE('',#14049,0.215) ;
#4974=CIRCLE('',#14051,0.215) ;
#4975=CIRCLE('',#14052,0.215) ;
#4976=CIRCLE('',#14054,0.51) ;
#4977=CIRCLE('',#14055,0.51) ;
#4978=CIRCLE('',#14057,10.) ;
#4979=CIRCLE('',#14058,10.) ;
#5681=VERTEX_POINT('',#20266) ;
#5682=VERTEX_POINT('',#20268) ;
#5683=VERTEX_POINT('',#20273) ;
#5684=VERTEX_POINT('',#20275) ;
#5685=VERTEX_POINT('',#20280) ;
#5686=VERTEX_POINT('',#20282) ;
#5687=VERTEX_POINT('',#20287) ;
#5688=VERTEX_POINT('',#20289) ;
#5689=VERTEX_POINT('',#20294) ;
#5690=VERTEX_POINT('',#20296) ;
#5691=VERTEX_POINT('',#20301) ;
#5692=VERTEX_POINT('',#20303) ;
#5693=VERTEX_POINT('',#20308) ;
#5694=VERTEX_POINT('',#20310) ;
#5695=VERTEX_POINT('',#20315) ;
#5696=VERTEX_POINT('',#20317) ;
#5697=VERTEX_POINT('',#20322) ;
#5698=VERTEX_POINT('',#20324) ;
#5699=VERTEX_POINT('',#20329) ;
#5700=VERTEX_POINT('',#20331) ;
#5701=VERTEX_POINT('',#20336) ;
#5702=VERTEX_POINT('',#20338) ;
#5703=VERTEX_POINT('',#20343) ;
#5704=VERTEX_POINT('',#20345) ;
#5705=VERTEX_POINT('',#20350) ;
#5706=VERTEX_POINT('',#20352) ;
#5707=VERTEX_POINT('',#20357) ;
#5708=VERTEX_POINT('',#20359) ;
#5709=VERTEX_POINT('',#20364) ;
#5710=VERTEX_POINT('',#20366) ;
#5711=VERTEX_POINT('',#20371) ;
#5712=VERTEX_POINT('',#20373) ;
#5713=VERTEX_POINT('',#20378) ;
#5714=VERTEX_POINT('',#20380) ;
#5715=VERTEX_POINT('',#20385) ;
#5716=VERTEX_POINT('',#20387) ;
#5717=VERTEX_POINT('',#20392) ;
#5718=VERTEX_POINT('',#20394) ;
#5719=VERTEX_POINT('',#20399) ;
#5720=VERTEX_POINT('',#20401) ;
#5721=VERTEX_POINT('',#20406) ;
#5722=VERTEX_POINT('',#20408) ;
#5723=VERTEX_POINT('',#20413) ;
#5724=VERTEX_POINT('',#20415) ;
#5725=VERTEX_POINT('',#20420) ;
#5726=VERTEX_POINT('',#20422) ;
#5727=VERTEX_POINT('',#20427) ;
#5728=VERTEX_POINT('',#20429) ;
#5729=VERTEX_POINT('',#20434) ;
#5730=VERTEX_POINT('',#20436) ;
#5731=VERTEX_POINT('',#20440) ;
#5732=VERTEX_POINT('',#20442) ;
#5733=VERTEX_POINT('',#20446) ;
#5734=VERTEX_POINT('',#20448) ;
#5735=VERTEX_POINT('',#20452) ;
#5736=VERTEX_POINT('',#20454) ;
#5737=VERTEX_POINT('',#20458) ;
#5738=VERTEX_POINT('',#20460) ;
#5739=VERTEX_POINT('',#20464) ;
#5740=VERTEX_POINT('',#20466) ;
#5741=VERTEX_POINT('',#20470) ;
#5742=VERTEX_POINT('',#20472) ;
#5743=VERTEX_POINT('',#20476) ;
#5744=VERTEX_POINT('',#20478) ;
#5745=VERTEX_POINT('',#20482) ;
#5746=VERTEX_POINT('',#20484) ;
#5747=VERTEX_POINT('',#20488) ;
#5748=VERTEX_POINT('',#20490) ;
#5749=VERTEX_POINT('',#20494) ;
#5750=VERTEX_POINT('',#20496) ;
#5751=VERTEX_POINT('',#20500) ;
#5752=VERTEX_POINT('',#20502) ;
#5753=VERTEX_POINT('',#20506) ;
#5754=VERTEX_POINT('',#20508) ;
#5755=VERTEX_POINT('',#20512) ;
#5756=VERTEX_POINT('',#20514) ;
#5757=VERTEX_POINT('',#20518) ;
#5758=VERTEX_POINT('',#20520) ;
#5759=VERTEX_POINT('',#20524) ;
#5760=VERTEX_POINT('',#20526) ;
#5761=VERTEX_POINT('',#20530) ;
#5762=VERTEX_POINT('',#20532) ;
#5763=VERTEX_POINT('',#20536) ;
#5764=VERTEX_POINT('',#20538) ;
#5765=VERTEX_POINT('',#20542) ;
#5766=VERTEX_POINT('',#20544) ;
#5767=VERTEX_POINT('',#20548) ;
#5768=VERTEX_POINT('',#20550) ;
#5769=VERTEX_POINT('',#20554) ;
#5770=VERTEX_POINT('',#20556) ;
#5771=VERTEX_POINT('',#20560) ;
#5772=VERTEX_POINT('',#20562) ;
#5773=VERTEX_POINT('',#20566) ;
#5774=VERTEX_POINT('',#20568) ;
#5775=VERTEX_POINT('',#20572) ;
#5776=VERTEX_POINT('',#20574) ;
#5777=VERTEX_POINT('',#20578) ;
#5778=VERTEX_POINT('',#20580) ;
#5779=VERTEX_POINT('',#20584) ;
#5780=VERTEX_POINT('',#20586) ;
#5781=VERTEX_POINT('',#20590) ;
#5782=VERTEX_POINT('',#20592) ;
#5783=VERTEX_POINT('',#20596) ;
#5784=VERTEX_POINT('',#20598) ;
#5785=VERTEX_POINT('',#20602) ;
#5786=VERTEX_POINT('',#20604) ;
#6949=EDGE_CURVE('',#5681,#5681,#4874,.T.) ;
#6950=EDGE_CURVE('',#5681,#5682,#1089,.T.) ;
#6951=EDGE_CURVE('',#5682,#5682,#4875,.T.) ;
#6952=EDGE_CURVE('',#5683,#5683,#4876,.T.) ;
#6953=EDGE_CURVE('',#5683,#5684,#1090,.T.) ;
#6954=EDGE_CURVE('',#5684,#5684,#4877,.T.) ;
#6955=EDGE_CURVE('',#5685,#5685,#4878,.T.) ;
#6956=EDGE_CURVE('',#5685,#5686,#1091,.T.) ;
#6957=EDGE_CURVE('',#5686,#5686,#4879,.T.) ;
#6958=EDGE_CURVE('',#5687,#5687,#4880,.T.) ;
#6959=EDGE_CURVE('',#5687,#5688,#1092,.T.) ;
#6960=EDGE_CURVE('',#5688,#5688,#4881,.T.) ;
#6961=EDGE_CURVE('',#5689,#5689,#4882,.T.) ;
#6962=EDGE_CURVE('',#5689,#5690,#1093,.T.) ;
#6963=EDGE_CURVE('',#5690,#5690,#4883,.T.) ;
#6964=EDGE_CURVE('',#5691,#5691,#4884,.T.) ;
#6965=EDGE_CURVE('',#5691,#5692,#1094,.T.) ;
#6966=EDGE_CURVE('',#5692,#5692,#4885,.T.) ;
#6967=EDGE_CURVE('',#5693,#5693,#4886,.T.) ;
#6968=EDGE_CURVE('',#5693,#5694,#1095,.T.) ;
#6969=EDGE_CURVE('',#5694,#5694,#4887,.T.) ;
#6970=EDGE_CURVE('',#5695,#5695,#4888,.T.) ;
#6971=EDGE_CURVE('',#5695,#5696,#1096,.T.) ;
#6972=EDGE_CURVE('',#5696,#5696,#4889,.T.) ;
#6973=EDGE_CURVE('',#5697,#5697,#4890,.T.) ;
#6974=EDGE_CURVE('',#5697,#5698,#1097,.T.) ;
#6975=EDGE_CURVE('',#5698,#5698,#4891,.T.) ;
#6976=EDGE_CURVE('',#5699,#5699,#4892,.T.) ;
#6977=EDGE_CURVE('',#5699,#5700,#1098,.T.) ;
#6978=EDGE_CURVE('',#5700,#5700,#4893,.T.) ;
#6979=EDGE_CURVE('',#5701,#5701,#4894,.T.) ;
#6980=EDGE_CURVE('',#5701,#5702,#1099,.T.) ;
#6981=EDGE_CURVE('',#5702,#5702,#4895,.T.) ;
#6982=EDGE_CURVE('',#5703,#5703,#4896,.T.) ;
#6983=EDGE_CURVE('',#5703,#5704,#1100,.T.) ;
#6984=EDGE_CURVE('',#5704,#5704,#4897,.T.) ;
#6985=EDGE_CURVE('',#5705,#5705,#4898,.T.) ;
#6986=EDGE_CURVE('',#5705,#5706,#1101,.T.) ;
#6987=EDGE_CURVE('',#5706,#5706,#4899,.T.) ;
#6988=EDGE_CURVE('',#5707,#5707,#4900,.T.) ;
#6989=EDGE_CURVE('',#5707,#5708,#1102,.T.) ;
#6990=EDGE_CURVE('',#5708,#5708,#4901,.T.) ;
#6991=EDGE_CURVE('',#5709,#5709,#4902,.T.) ;
#6992=EDGE_CURVE('',#5709,#5710,#1103,.T.) ;
#6993=EDGE_CURVE('',#5710,#5710,#4903,.T.) ;
#6994=EDGE_CURVE('',#5711,#5711,#4904,.T.) ;
#6995=EDGE_CURVE('',#5711,#5712,#1104,.T.) ;
#6996=EDGE_CURVE('',#5712,#5712,#4905,.T.) ;
#6997=EDGE_CURVE('',#5713,#5713,#4906,.T.) ;
#6998=EDGE_CURVE('',#5713,#5714,#1105,.T.) ;
#6999=EDGE_CURVE('',#5714,#5714,#4907,.T.) ;
#7000=EDGE_CURVE('',#5715,#5715,#4908,.T.) ;
#7001=EDGE_CURVE('',#5715,#5716,#1106,.T.) ;
#7002=EDGE_CURVE('',#5716,#5716,#4909,.T.) ;
#7003=EDGE_CURVE('',#5717,#5717,#4910,.T.) ;
#7004=EDGE_CURVE('',#5717,#5718,#1107,.T.) ;
#7005=EDGE_CURVE('',#5718,#5718,#4911,.T.) ;
#7006=EDGE_CURVE('',#5719,#5719,#4912,.T.) ;
#7007=EDGE_CURVE('',#5719,#5720,#1108,.T.) ;
#7008=EDGE_CURVE('',#5720,#5720,#4913,.T.) ;
#7009=EDGE_CURVE('',#5721,#5721,#4914,.T.) ;
#7010=EDGE_CURVE('',#5721,#5722,#1109,.T.) ;
#7011=EDGE_CURVE('',#5722,#5722,#4915,.T.) ;
#7012=EDGE_CURVE('',#5723,#5723,#4916,.T.) ;
#7013=EDGE_CURVE('',#5723,#5724,#1110,.T.) ;
#7014=EDGE_CURVE('',#5724,#5724,#4917,.T.) ;
#7015=EDGE_CURVE('',#5725,#5725,#4918,.T.) ;
#7016=EDGE_CURVE('',#5725,#5726,#1111,.T.) ;
#7017=EDGE_CURVE('',#5726,#5726,#4919,.T.) ;
#7018=EDGE_CURVE('',#5727,#5727,#4920,.T.) ;
#7019=EDGE_CURVE('',#5727,#5728,#1112,.T.) ;
#7020=EDGE_CURVE('',#5728,#5728,#4921,.T.) ;
#7021=EDGE_CURVE('',#5729,#5729,#4922,.T.) ;
#7022=EDGE_CURVE('',#5729,#5730,#1113,.T.) ;
#7023=EDGE_CURVE('',#5730,#5730,#4923,.T.) ;
#7024=EDGE_CURVE('',#5731,#5731,#4924,.T.) ;
#7025=EDGE_CURVE('',#5731,#5732,#1114,.T.) ;
#7026=EDGE_CURVE('',#5732,#5732,#4925,.T.) ;
#7027=EDGE_CURVE('',#5733,#5733,#4926,.T.) ;
#7028=EDGE_CURVE('',#5733,#5734,#1115,.T.) ;
#7029=EDGE_CURVE('',#5734,#5734,#4927,.T.) ;
#7030=EDGE_CURVE('',#5735,#5735,#4928,.T.) ;
#7031=EDGE_CURVE('',#5735,#5736,#1116,.T.) ;
#7032=EDGE_CURVE('',#5736,#5736,#4929,.T.) ;
#7033=EDGE_CURVE('',#5737,#5737,#4930,.T.) ;
#7034=EDGE_CURVE('',#5737,#5738,#1117,.T.) ;
#7035=EDGE_CURVE('',#5738,#5738,#4931,.T.) ;
#7036=EDGE_CURVE('',#5739,#5739,#4932,.T.) ;
#7037=EDGE_CURVE('',#5739,#5740,#1118,.T.) ;
#7038=EDGE_CURVE('',#5740,#5740,#4933,.T.) ;
#7039=EDGE_CURVE('',#5741,#5741,#4934,.T.) ;
#7040=EDGE_CURVE('',#5741,#5742,#1119,.T.) ;
#7041=EDGE_CURVE('',#5742,#5742,#4935,.T.) ;
#7042=EDGE_CURVE('',#5743,#5743,#4936,.T.) ;
#7043=EDGE_CURVE('',#5743,#5744,#1120,.T.) ;
#7044=EDGE_CURVE('',#5744,#5744,#4937,.T.) ;
#7045=EDGE_CURVE('',#5745,#5745,#4938,.T.) ;
#7046=EDGE_CURVE('',#5745,#5746,#1121,.T.) ;
#7047=EDGE_CURVE('',#5746,#5746,#4939,.T.) ;
#7048=EDGE_CURVE('',#5747,#5747,#4940,.T.) ;
#7049=EDGE_CURVE('',#5747,#5748,#1122,.T.) ;
#7050=EDGE_CURVE('',#5748,#5748,#4941,.T.) ;
#7051=EDGE_CURVE('',#5749,#5749,#4942,.T.) ;
#7052=EDGE_CURVE('',#5749,#5750,#1123,.T.) ;
#7053=EDGE_CURVE('',#5750,#5750,#4943,.T.) ;
#7054=EDGE_CURVE('',#5751,#5751,#4944,.T.) ;
#7055=EDGE_CURVE('',#5751,#5752,#1124,.T.) ;
#7056=EDGE_CURVE('',#5752,#5752,#4945,.T.) ;
#7057=EDGE_CURVE('',#5753,#5753,#4946,.T.) ;
#7058=EDGE_CURVE('',#5753,#5754,#1125,.T.) ;
#7059=EDGE_CURVE('',#5754,#5754,#4947,.T.) ;
#7060=EDGE_CURVE('',#5755,#5755,#4948,.T.) ;
#7061=EDGE_CURVE('',#5755,#5756,#1126,.T.) ;
#7062=EDGE_CURVE('',#5756,#5756,#4949,.T.) ;
#7063=EDGE_CURVE('',#5757,#5757,#4950,.T.) ;
#7064=EDGE_CURVE('',#5757,#5758,#1127,.T.) ;
#7065=EDGE_CURVE('',#5758,#5758,#4951,.T.) ;
#7066=EDGE_CURVE('',#5759,#5759,#4952,.T.) ;
#7067=EDGE_CURVE('',#5759,#5760,#1128,.T.) ;
#7068=EDGE_CURVE('',#5760,#5760,#4953,.T.) ;
#7069=EDGE_CURVE('',#5761,#5761,#4954,.T.) ;
#7070=EDGE_CURVE('',#5761,#5762,#1129,.T.) ;
#7071=EDGE_CURVE('',#5762,#5762,#4955,.T.) ;
#7072=EDGE_CURVE('',#5763,#5763,#4956,.T.) ;
#7073=EDGE_CURVE('',#5763,#5764,#1130,.T.) ;
#7074=EDGE_CURVE('',#5764,#5764,#4957,.T.) ;
#7075=EDGE_CURVE('',#5765,#5765,#4958,.T.) ;
#7076=EDGE_CURVE('',#5765,#5766,#1131,.T.) ;
#7077=EDGE_CURVE('',#5766,#5766,#4959,.T.) ;
#7078=EDGE_CURVE('',#5767,#5767,#4960,.T.) ;
#7079=EDGE_CURVE('',#5767,#5768,#1132,.T.) ;
#7080=EDGE_CURVE('',#5768,#5768,#4961,.T.) ;
#7081=EDGE_CURVE('',#5769,#5769,#4962,.T.) ;
#7082=EDGE_CURVE('',#5769,#5770,#1133,.T.) ;
#7083=EDGE_CURVE('',#5770,#5770,#4963,.T.) ;
#7084=EDGE_CURVE('',#5771,#5771,#4964,.T.) ;
#7085=EDGE_CURVE('',#5771,#5772,#1134,.T.) ;
#7086=EDGE_CURVE('',#5772,#5772,#4965,.T.) ;
#7087=EDGE_CURVE('',#5773,#5773,#4966,.T.) ;
#7088=EDGE_CURVE('',#5773,#5774,#1135,.T.) ;
#7089=EDGE_CURVE('',#5774,#5774,#4967,.T.) ;
#7090=EDGE_CURVE('',#5775,#5775,#4968,.T.) ;
#7091=EDGE_CURVE('',#5775,#5776,#1136,.T.) ;
#7092=EDGE_CURVE('',#5776,#5776,#4969,.T.) ;
#7093=EDGE_CURVE('',#5777,#5777,#4970,.T.) ;
#7094=EDGE_CURVE('',#5777,#5778,#1137,.T.) ;
#7095=EDGE_CURVE('',#5778,#5778,#4971,.T.) ;
#7096=EDGE_CURVE('',#5779,#5779,#4972,.T.) ;
#7097=EDGE_CURVE('',#5779,#5780,#1138,.T.) ;
#7098=EDGE_CURVE('',#5780,#5780,#4973,.T.) ;
#7099=EDGE_CURVE('',#5781,#5781,#4974,.T.) ;
#7100=EDGE_CURVE('',#5781,#5782,#1139,.T.) ;
#7101=EDGE_CURVE('',#5782,#5782,#4975,.T.) ;
#7102=EDGE_CURVE('',#5783,#5783,#4976,.T.) ;
#7103=EDGE_CURVE('',#5783,#5784,#1140,.T.) ;
#7104=EDGE_CURVE('',#5784,#5784,#4977,.T.) ;
#7105=EDGE_CURVE('',#5785,#5785,#4978,.T.) ;
#7106=EDGE_CURVE('',#5785,#5786,#1141,.T.) ;
#7107=EDGE_CURVE('',#5786,#5786,#4979,.T.) ;
#8919=ORIENTED_EDGE('',*,*,#6949,.F.) ;
#8920=ORIENTED_EDGE('',*,*,#6950,.T.) ;
#8921=ORIENTED_EDGE('',*,*,#6951,.T.) ;
#8922=ORIENTED_EDGE('',*,*,#6950,.F.) ;
#8923=ORIENTED_EDGE('',*,*,#6951,.F.) ;
#8924=ORIENTED_EDGE('',*,*,#6952,.F.) ;
#8925=ORIENTED_EDGE('',*,*,#6953,.T.) ;
#8926=ORIENTED_EDGE('',*,*,#6954,.T.) ;
#8927=ORIENTED_EDGE('',*,*,#6953,.F.) ;
#8928=ORIENTED_EDGE('',*,*,#6954,.F.) ;
#8929=ORIENTED_EDGE('',*,*,#6955,.F.) ;
#8930=ORIENTED_EDGE('',*,*,#6956,.T.) ;
#8931=ORIENTED_EDGE('',*,*,#6957,.T.) ;
#8932=ORIENTED_EDGE('',*,*,#6956,.F.) ;
#8933=ORIENTED_EDGE('',*,*,#6957,.F.) ;
#8934=ORIENTED_EDGE('',*,*,#6958,.F.) ;
#8935=ORIENTED_EDGE('',*,*,#6959,.T.) ;
#8936=ORIENTED_EDGE('',*,*,#6960,.T.) ;
#8937=ORIENTED_EDGE('',*,*,#6959,.F.) ;
#8938=ORIENTED_EDGE('',*,*,#6960,.F.) ;
#8939=ORIENTED_EDGE('',*,*,#6961,.F.) ;
#8940=ORIENTED_EDGE('',*,*,#6962,.T.) ;
#8941=ORIENTED_EDGE('',*,*,#6963,.T.) ;
#8942=ORIENTED_EDGE('',*,*,#6962,.F.) ;
#8943=ORIENTED_EDGE('',*,*,#6963,.F.) ;
#8944=ORIENTED_EDGE('',*,*,#6964,.F.) ;
#8945=ORIENTED_EDGE('',*,*,#6965,.T.) ;
#8946=ORIENTED_EDGE('',*,*,#6966,.T.) ;
#8947=ORIENTED_EDGE('',*,*,#6965,.F.) ;
#8948=ORIENTED_EDGE('',*,*,#6966,.F.) ;
#8949=ORIENTED_EDGE('',*,*,#6967,.F.) ;
#8950=ORIENTED_EDGE('',*,*,#6968,.T.) ;
#8951=ORIENTED_EDGE('',*,*,#6969,.T.) ;
#8952=ORIENTED_EDGE('',*,*,#6968,.F.) ;
#8953=ORIENTED_EDGE('',*,*,#6969,.F.) ;
#8954=ORIENTED_EDGE('',*,*,#6970,.F.) ;
#8955=ORIENTED_EDGE('',*,*,#6971,.T.) ;
#8956=ORIENTED_EDGE('',*,*,#6972,.T.) ;
#8957=ORIENTED_EDGE('',*,*,#6971,.F.) ;
#8958=ORIENTED_EDGE('',*,*,#6972,.F.) ;
#8959=ORIENTED_EDGE('',*,*,#6973,.F.) ;
#8960=ORIENTED_EDGE('',*,*,#6974,.T.) ;
#8961=ORIENTED_EDGE('',*,*,#6975,.T.) ;
#8962=ORIENTED_EDGE('',*,*,#6974,.F.) ;
#8963=ORIENTED_EDGE('',*,*,#6975,.F.) ;
#8964=ORIENTED_EDGE('',*,*,#6976,.F.) ;
#8965=ORIENTED_EDGE('',*,*,#6977,.T.) ;
#8966=ORIENTED_EDGE('',*,*,#6978,.T.) ;
#8967=ORIENTED_EDGE('',*,*,#6977,.F.) ;
#8968=ORIENTED_EDGE('',*,*,#6978,.F.) ;
#8969=ORIENTED_EDGE('',*,*,#6979,.F.) ;
#8970=ORIENTED_EDGE('',*,*,#6980,.T.) ;
#8971=ORIENTED_EDGE('',*,*,#6981,.T.) ;
#8972=ORIENTED_EDGE('',*,*,#6980,.F.) ;
#8973=ORIENTED_EDGE('',*,*,#6981,.F.) ;
#8974=ORIENTED_EDGE('',*,*,#6982,.F.) ;
#8975=ORIENTED_EDGE('',*,*,#6983,.T.) ;
#8976=ORIENTED_EDGE('',*,*,#6984,.T.) ;
#8977=ORIENTED_EDGE('',*,*,#6983,.F.) ;
#8978=ORIENTED_EDGE('',*,*,#6984,.F.) ;
#8979=ORIENTED_EDGE('',*,*,#6985,.F.) ;
#8980=ORIENTED_EDGE('',*,*,#6986,.T.) ;
#8981=ORIENTED_EDGE('',*,*,#6987,.T.) ;
#8982=ORIENTED_EDGE('',*,*,#6986,.F.) ;
#8983=ORIENTED_EDGE('',*,*,#6987,.F.) ;
#8984=ORIENTED_EDGE('',*,*,#6988,.F.) ;
#8985=ORIENTED_EDGE('',*,*,#6989,.T.) ;
#8986=ORIENTED_EDGE('',*,*,#6990,.T.) ;
#8987=ORIENTED_EDGE('',*,*,#6989,.F.) ;
#8988=ORIENTED_EDGE('',*,*,#6990,.F.) ;
#8989=ORIENTED_EDGE('',*,*,#6991,.F.) ;
#8990=ORIENTED_EDGE('',*,*,#6992,.T.) ;
#8991=ORIENTED_EDGE('',*,*,#6993,.T.) ;
#8992=ORIENTED_EDGE('',*,*,#6992,.F.) ;
#8993=ORIENTED_EDGE('',*,*,#6993,.F.) ;
#8994=ORIENTED_EDGE('',*,*,#6994,.F.) ;
#8995=ORIENTED_EDGE('',*,*,#6995,.T.) ;
#8996=ORIENTED_EDGE('',*,*,#6996,.T.) ;
#8997=ORIENTED_EDGE('',*,*,#6995,.F.) ;
#8998=ORIENTED_EDGE('',*,*,#6996,.F.) ;
#8999=ORIENTED_EDGE('',*,*,#6997,.F.) ;
#9000=ORIENTED_EDGE('',*,*,#6998,.T.) ;
#9001=ORIENTED_EDGE('',*,*,#6999,.T.) ;
#9002=ORIENTED_EDGE('',*,*,#6998,.F.) ;
#9003=ORIENTED_EDGE('',*,*,#6999,.F.) ;
#9004=ORIENTED_EDGE('',*,*,#7000,.F.) ;
#9005=ORIENTED_EDGE('',*,*,#7001,.T.) ;
#9006=ORIENTED_EDGE('',*,*,#7002,.T.) ;
#9007=ORIENTED_EDGE('',*,*,#7001,.F.) ;
#9008=ORIENTED_EDGE('',*,*,#7002,.F.) ;
#9009=ORIENTED_EDGE('',*,*,#7003,.F.) ;
#9010=ORIENTED_EDGE('',*,*,#7004,.T.) ;
#9011=ORIENTED_EDGE('',*,*,#7005,.T.) ;
#9012=ORIENTED_EDGE('',*,*,#7004,.F.) ;
#9013=ORIENTED_EDGE('',*,*,#7005,.F.) ;
#9014=ORIENTED_EDGE('',*,*,#7006,.F.) ;
#9015=ORIENTED_EDGE('',*,*,#7007,.T.) ;
#9016=ORIENTED_EDGE('',*,*,#7008,.T.) ;
#9017=ORIENTED_EDGE('',*,*,#7007,.F.) ;
#9018=ORIENTED_EDGE('',*,*,#7008,.F.) ;
#9019=ORIENTED_EDGE('',*,*,#7009,.F.) ;
#9020=ORIENTED_EDGE('',*,*,#7010,.T.) ;
#9021=ORIENTED_EDGE('',*,*,#7011,.T.) ;
#9022=ORIENTED_EDGE('',*,*,#7010,.F.) ;
#9023=ORIENTED_EDGE('',*,*,#7011,.F.) ;
#9024=ORIENTED_EDGE('',*,*,#7012,.F.) ;
#9025=ORIENTED_EDGE('',*,*,#7013,.T.) ;
#9026=ORIENTED_EDGE('',*,*,#7014,.T.) ;
#9027=ORIENTED_EDGE('',*,*,#7013,.F.) ;
#9028=ORIENTED_EDGE('',*,*,#7014,.F.) ;
#9029=ORIENTED_EDGE('',*,*,#7015,.F.) ;
#9030=ORIENTED_EDGE('',*,*,#7016,.T.) ;
#9031=ORIENTED_EDGE('',*,*,#7017,.T.) ;
#9032=ORIENTED_EDGE('',*,*,#7016,.F.) ;
#9033=ORIENTED_EDGE('',*,*,#7017,.F.) ;
#9034=ORIENTED_EDGE('',*,*,#7018,.F.) ;
#9035=ORIENTED_EDGE('',*,*,#7019,.T.) ;
#9036=ORIENTED_EDGE('',*,*,#7020,.T.) ;
#9037=ORIENTED_EDGE('',*,*,#7019,.F.) ;
#9038=ORIENTED_EDGE('',*,*,#7020,.F.) ;
#9039=ORIENTED_EDGE('',*,*,#7021,.F.) ;
#9040=ORIENTED_EDGE('',*,*,#7022,.T.) ;
#9041=ORIENTED_EDGE('',*,*,#7023,.F.) ;
#9042=ORIENTED_EDGE('',*,*,#7022,.F.) ;
#9043=ORIENTED_EDGE('',*,*,#7024,.F.) ;
#9044=ORIENTED_EDGE('',*,*,#7025,.T.) ;
#9045=ORIENTED_EDGE('',*,*,#7026,.F.) ;
#9046=ORIENTED_EDGE('',*,*,#7025,.F.) ;
#9047=ORIENTED_EDGE('',*,*,#7027,.F.) ;
#9048=ORIENTED_EDGE('',*,*,#7028,.T.) ;
#9049=ORIENTED_EDGE('',*,*,#7029,.F.) ;
#9050=ORIENTED_EDGE('',*,*,#7028,.F.) ;
#9051=ORIENTED_EDGE('',*,*,#7030,.F.) ;
#9052=ORIENTED_EDGE('',*,*,#7031,.T.) ;
#9053=ORIENTED_EDGE('',*,*,#7032,.F.) ;
#9054=ORIENTED_EDGE('',*,*,#7031,.F.) ;
#9055=ORIENTED_EDGE('',*,*,#7033,.F.) ;
#9056=ORIENTED_EDGE('',*,*,#7034,.T.) ;
#9057=ORIENTED_EDGE('',*,*,#7035,.F.) ;
#9058=ORIENTED_EDGE('',*,*,#7034,.F.) ;
#9059=ORIENTED_EDGE('',*,*,#7036,.F.) ;
#9060=ORIENTED_EDGE('',*,*,#7037,.T.) ;
#9061=ORIENTED_EDGE('',*,*,#7038,.F.) ;
#9062=ORIENTED_EDGE('',*,*,#7037,.F.) ;
#9063=ORIENTED_EDGE('',*,*,#7039,.F.) ;
#9064=ORIENTED_EDGE('',*,*,#7040,.T.) ;
#9065=ORIENTED_EDGE('',*,*,#7041,.F.) ;
#9066=ORIENTED_EDGE('',*,*,#7040,.F.) ;
#9067=ORIENTED_EDGE('',*,*,#7042,.F.) ;
#9068=ORIENTED_EDGE('',*,*,#7043,.T.) ;
#9069=ORIENTED_EDGE('',*,*,#7044,.F.) ;
#9070=ORIENTED_EDGE('',*,*,#7043,.F.) ;
#9071=ORIENTED_EDGE('',*,*,#7045,.F.) ;
#9072=ORIENTED_EDGE('',*,*,#7046,.T.) ;
#9073=ORIENTED_EDGE('',*,*,#7047,.F.) ;
#9074=ORIENTED_EDGE('',*,*,#7046,.F.) ;
#9075=ORIENTED_EDGE('',*,*,#7048,.F.) ;
#9076=ORIENTED_EDGE('',*,*,#7049,.T.) ;
#9077=ORIENTED_EDGE('',*,*,#7050,.F.) ;
#9078=ORIENTED_EDGE('',*,*,#7049,.F.) ;
#9079=ORIENTED_EDGE('',*,*,#7051,.F.) ;
#9080=ORIENTED_EDGE('',*,*,#7052,.T.) ;
#9081=ORIENTED_EDGE('',*,*,#7053,.F.) ;
#9082=ORIENTED_EDGE('',*,*,#7052,.F.) ;
#9083=ORIENTED_EDGE('',*,*,#7054,.F.) ;
#9084=ORIENTED_EDGE('',*,*,#7055,.T.) ;
#9085=ORIENTED_EDGE('',*,*,#7056,.F.) ;
#9086=ORIENTED_EDGE('',*,*,#7055,.F.) ;
#9087=ORIENTED_EDGE('',*,*,#7057,.F.) ;
#9088=ORIENTED_EDGE('',*,*,#7058,.T.) ;
#9089=ORIENTED_EDGE('',*,*,#7059,.F.) ;
#9090=ORIENTED_EDGE('',*,*,#7058,.F.) ;
#9091=ORIENTED_EDGE('',*,*,#7060,.F.) ;
#9092=ORIENTED_EDGE('',*,*,#7061,.T.) ;
#9093=ORIENTED_EDGE('',*,*,#7062,.F.) ;
#9094=ORIENTED_EDGE('',*,*,#7061,.F.) ;
#9095=ORIENTED_EDGE('',*,*,#7063,.F.) ;
#9096=ORIENTED_EDGE('',*,*,#7064,.T.) ;
#9097=ORIENTED_EDGE('',*,*,#7065,.F.) ;
#9098=ORIENTED_EDGE('',*,*,#7064,.F.) ;
#9099=ORIENTED_EDGE('',*,*,#7066,.F.) ;
#9100=ORIENTED_EDGE('',*,*,#7067,.T.) ;
#9101=ORIENTED_EDGE('',*,*,#7068,.F.) ;
#9102=ORIENTED_EDGE('',*,*,#7067,.F.) ;
#9103=ORIENTED_EDGE('',*,*,#7069,.F.) ;
#9104=ORIENTED_EDGE('',*,*,#7070,.T.) ;
#9105=ORIENTED_EDGE('',*,*,#7071,.F.) ;
#9106=ORIENTED_EDGE('',*,*,#7070,.F.) ;
#9107=ORIENTED_EDGE('',*,*,#7072,.F.) ;
#9108=ORIENTED_EDGE('',*,*,#7073,.T.) ;
#9109=ORIENTED_EDGE('',*,*,#7074,.F.) ;
#9110=ORIENTED_EDGE('',*,*,#7073,.F.) ;
#9111=ORIENTED_EDGE('',*,*,#7075,.F.) ;
#9112=ORIENTED_EDGE('',*,*,#7076,.T.) ;
#9113=ORIENTED_EDGE('',*,*,#7077,.F.) ;
#9114=ORIENTED_EDGE('',*,*,#7076,.F.) ;
#9115=ORIENTED_EDGE('',*,*,#7078,.F.) ;
#9116=ORIENTED_EDGE('',*,*,#7079,.T.) ;
#9117=ORIENTED_EDGE('',*,*,#7080,.F.) ;
#9118=ORIENTED_EDGE('',*,*,#7079,.F.) ;
#9119=ORIENTED_EDGE('',*,*,#7081,.F.) ;
#9120=ORIENTED_EDGE('',*,*,#7082,.T.) ;
#9121=ORIENTED_EDGE('',*,*,#7083,.F.) ;
#9122=ORIENTED_EDGE('',*,*,#7082,.F.) ;
#9123=ORIENTED_EDGE('',*,*,#7084,.F.) ;
#9124=ORIENTED_EDGE('',*,*,#7085,.T.) ;
#9125=ORIENTED_EDGE('',*,*,#7086,.F.) ;
#9126=ORIENTED_EDGE('',*,*,#7085,.F.) ;
#9127=ORIENTED_EDGE('',*,*,#7087,.F.) ;
#9128=ORIENTED_EDGE('',*,*,#7088,.T.) ;
#9129=ORIENTED_EDGE('',*,*,#7089,.F.) ;
#9130=ORIENTED_EDGE('',*,*,#7088,.F.) ;
#9131=ORIENTED_EDGE('',*,*,#7090,.F.) ;
#9132=ORIENTED_EDGE('',*,*,#7091,.T.) ;
#9133=ORIENTED_EDGE('',*,*,#7092,.F.) ;
#9134=ORIENTED_EDGE('',*,*,#7091,.F.) ;
#9135=ORIENTED_EDGE('',*,*,#7093,.F.) ;
#9136=ORIENTED_EDGE('',*,*,#7094,.T.) ;
#9137=ORIENTED_EDGE('',*,*,#7095,.F.) ;
#9138=ORIENTED_EDGE('',*,*,#7094,.F.) ;
#9139=ORIENTED_EDGE('',*,*,#7096,.F.) ;
#9140=ORIENTED_EDGE('',*,*,#7097,.T.) ;
#9141=ORIENTED_EDGE('',*,*,#7098,.F.) ;
#9142=ORIENTED_EDGE('',*,*,#7097,.F.) ;
#9143=ORIENTED_EDGE('',*,*,#7099,.F.) ;
#9144=ORIENTED_EDGE('',*,*,#7100,.T.) ;
#9145=ORIENTED_EDGE('',*,*,#7101,.F.) ;
#9146=ORIENTED_EDGE('',*,*,#7100,.F.) ;
#9147=ORIENTED_EDGE('',*,*,#7102,.F.) ;
#9148=ORIENTED_EDGE('',*,*,#7103,.T.) ;
#9149=ORIENTED_EDGE('',*,*,#7104,.F.) ;
#9150=ORIENTED_EDGE('',*,*,#7103,.F.) ;
#9151=ORIENTED_EDGE('',*,*,#7105,.F.) ;
#9152=ORIENTED_EDGE('',*,*,#7106,.T.) ;
#9153=ORIENTED_EDGE('',*,*,#7107,.F.) ;
#9154=ORIENTED_EDGE('',*,*,#7106,.F.) ;
#9155=ORIENTED_EDGE('',*,*,#7107,.T.) ;
#9156=ORIENTED_EDGE('',*,*,#6952,.T.) ;
#9157=ORIENTED_EDGE('',*,*,#6958,.T.) ;
#9158=ORIENTED_EDGE('',*,*,#6964,.T.) ;
#9159=ORIENTED_EDGE('',*,*,#6970,.T.) ;
#9160=ORIENTED_EDGE('',*,*,#6976,.T.) ;
#9161=ORIENTED_EDGE('',*,*,#6982,.T.) ;
#9162=ORIENTED_EDGE('',*,*,#6988,.T.) ;
#9163=ORIENTED_EDGE('',*,*,#6994,.T.) ;
#9164=ORIENTED_EDGE('',*,*,#7000,.T.) ;
#9165=ORIENTED_EDGE('',*,*,#7006,.T.) ;
#9166=ORIENTED_EDGE('',*,*,#7012,.T.) ;
#9167=ORIENTED_EDGE('',*,*,#7018,.T.) ;
#9168=ORIENTED_EDGE('',*,*,#7024,.T.) ;
#9169=ORIENTED_EDGE('',*,*,#7030,.T.) ;
#9170=ORIENTED_EDGE('',*,*,#7036,.T.) ;
#9171=ORIENTED_EDGE('',*,*,#7042,.T.) ;
#9172=ORIENTED_EDGE('',*,*,#7048,.T.) ;
#9173=ORIENTED_EDGE('',*,*,#7054,.T.) ;
#9174=ORIENTED_EDGE('',*,*,#7060,.T.) ;
#9175=ORIENTED_EDGE('',*,*,#7066,.T.) ;
#9176=ORIENTED_EDGE('',*,*,#7072,.T.) ;
#9177=ORIENTED_EDGE('',*,*,#7078,.T.) ;
#9178=ORIENTED_EDGE('',*,*,#7102,.T.) ;
#9179=ORIENTED_EDGE('',*,*,#7099,.T.) ;
#9180=ORIENTED_EDGE('',*,*,#7096,.T.) ;
#9181=ORIENTED_EDGE('',*,*,#7093,.T.) ;
#9182=ORIENTED_EDGE('',*,*,#7090,.T.) ;
#9183=ORIENTED_EDGE('',*,*,#7087,.T.) ;
#9184=ORIENTED_EDGE('',*,*,#7084,.T.) ;
#9185=ORIENTED_EDGE('',*,*,#7081,.T.) ;
#9186=ORIENTED_EDGE('',*,*,#7075,.T.) ;
#9187=ORIENTED_EDGE('',*,*,#7069,.T.) ;
#9188=ORIENTED_EDGE('',*,*,#7063,.T.) ;
#9189=ORIENTED_EDGE('',*,*,#7057,.T.) ;
#9190=ORIENTED_EDGE('',*,*,#7051,.T.) ;
#9191=ORIENTED_EDGE('',*,*,#7045,.T.) ;
#9192=ORIENTED_EDGE('',*,*,#7039,.T.) ;
#9193=ORIENTED_EDGE('',*,*,#7033,.T.) ;
#9194=ORIENTED_EDGE('',*,*,#7027,.T.) ;
#9195=ORIENTED_EDGE('',*,*,#7021,.T.) ;
#9196=ORIENTED_EDGE('',*,*,#7015,.T.) ;
#9197=ORIENTED_EDGE('',*,*,#7009,.T.) ;
#9198=ORIENTED_EDGE('',*,*,#7003,.T.) ;
#9199=ORIENTED_EDGE('',*,*,#6997,.T.) ;
#9200=ORIENTED_EDGE('',*,*,#6991,.T.) ;
#9201=ORIENTED_EDGE('',*,*,#6985,.T.) ;
#9202=ORIENTED_EDGE('',*,*,#6979,.T.) ;
#9203=ORIENTED_EDGE('',*,*,#6973,.T.) ;
#9204=ORIENTED_EDGE('',*,*,#6967,.T.) ;
#9205=ORIENTED_EDGE('',*,*,#6961,.T.) ;
#9206=ORIENTED_EDGE('',*,*,#6955,.T.) ;
#9207=ORIENTED_EDGE('',*,*,#6949,.T.) ;
#9208=ORIENTED_EDGE('',*,*,#7105,.T.) ;
#9209=ORIENTED_EDGE('',*,*,#7026,.T.) ;
#9210=ORIENTED_EDGE('',*,*,#7032,.T.) ;
#9211=ORIENTED_EDGE('',*,*,#7038,.T.) ;
#9212=ORIENTED_EDGE('',*,*,#7044,.T.) ;
#9213=ORIENTED_EDGE('',*,*,#7050,.T.) ;
#9214=ORIENTED_EDGE('',*,*,#7056,.T.) ;
#9215=ORIENTED_EDGE('',*,*,#7062,.T.) ;
#9216=ORIENTED_EDGE('',*,*,#7068,.T.) ;
#9217=ORIENTED_EDGE('',*,*,#7074,.T.) ;
#9218=ORIENTED_EDGE('',*,*,#7080,.T.) ;
#9219=ORIENTED_EDGE('',*,*,#7104,.T.) ;
#9220=ORIENTED_EDGE('',*,*,#7101,.T.) ;
#9221=ORIENTED_EDGE('',*,*,#7098,.T.) ;
#9222=ORIENTED_EDGE('',*,*,#7095,.T.) ;
#9223=ORIENTED_EDGE('',*,*,#7092,.T.) ;
#9224=ORIENTED_EDGE('',*,*,#7089,.T.) ;
#9225=ORIENTED_EDGE('',*,*,#7086,.T.) ;
#9226=ORIENTED_EDGE('',*,*,#7083,.T.) ;
#9227=ORIENTED_EDGE('',*,*,#7077,.T.) ;
#9228=ORIENTED_EDGE('',*,*,#7071,.T.) ;
#9229=ORIENTED_EDGE('',*,*,#7065,.T.) ;
#9230=ORIENTED_EDGE('',*,*,#7059,.T.) ;
#9231=ORIENTED_EDGE('',*,*,#7053,.T.) ;
#9232=ORIENTED_EDGE('',*,*,#7047,.T.) ;
#9233=ORIENTED_EDGE('',*,*,#7041,.T.) ;
#9234=ORIENTED_EDGE('',*,*,#7035,.T.) ;
#9235=ORIENTED_EDGE('',*,*,#7029,.T.) ;
#9236=ORIENTED_EDGE('',*,*,#7023,.T.) ;
#12036=PLANE('',#13879) ;
#12037=PLANE('',#13883) ;
#12038=PLANE('',#13887) ;
#12039=PLANE('',#13891) ;
#12040=PLANE('',#13895) ;
#12041=PLANE('',#13899) ;
#12042=PLANE('',#13903) ;
#12043=PLANE('',#13907) ;
#12044=PLANE('',#13911) ;
#12045=PLANE('',#13915) ;
#12046=PLANE('',#13919) ;
#12047=PLANE('',#13923) ;
#12048=PLANE('',#13927) ;
#12049=PLANE('',#13931) ;
#12050=PLANE('',#13935) ;
#12051=PLANE('',#13939) ;
#12052=PLANE('',#13943) ;
#12053=PLANE('',#13947) ;
#12054=PLANE('',#13951) ;
#12055=PLANE('',#13955) ;
#12056=PLANE('',#13959) ;
#12057=PLANE('',#13963) ;
#12058=PLANE('',#13967) ;
#12059=PLANE('',#13971) ;
#12060=PLANE('',#14059) ;
#12061=PLANE('',#14060) ;
#12440=ADVANCED_FACE('',(#3045),#2725,.F.) ;
#12441=ADVANCED_FACE('',(#3046),#12036,.F.) ;
#12442=ADVANCED_FACE('',(#3047),#2726,.F.) ;
#12443=ADVANCED_FACE('',(#3048),#12037,.F.) ;
#12444=ADVANCED_FACE('',(#3049),#2727,.F.) ;
#12445=ADVANCED_FACE('',(#3050),#12038,.F.) ;
#12446=ADVANCED_FACE('',(#3051),#2728,.F.) ;
#12447=ADVANCED_FACE('',(#3052),#12039,.F.) ;
#12448=ADVANCED_FACE('',(#3053),#2729,.F.) ;
#12449=ADVANCED_FACE('',(#3054),#12040,.F.) ;
#12450=ADVANCED_FACE('',(#3055),#2730,.F.) ;
#12451=ADVANCED_FACE('',(#3056),#12041,.F.) ;
#12452=ADVANCED_FACE('',(#3057),#2731,.F.) ;
#12453=ADVANCED_FACE('',(#3058),#12042,.F.) ;
#12454=ADVANCED_FACE('',(#3059),#2732,.F.) ;
#12455=ADVANCED_FACE('',(#3060),#12043,.F.) ;
#12456=ADVANCED_FACE('',(#3061),#2733,.F.) ;
#12457=ADVANCED_FACE('',(#3062),#12044,.F.) ;
#12458=ADVANCED_FACE('',(#3063),#2734,.F.) ;
#12459=ADVANCED_FACE('',(#3064),#12045,.F.) ;
#12460=ADVANCED_FACE('',(#3065),#2735,.F.) ;
#12461=ADVANCED_FACE('',(#3066),#12046,.F.) ;
#12462=ADVANCED_FACE('',(#3067),#2736,.F.) ;
#12463=ADVANCED_FACE('',(#3068),#12047,.F.) ;
#12464=ADVANCED_FACE('',(#3069),#2737,.F.) ;
#12465=ADVANCED_FACE('',(#3070),#12048,.F.) ;
#12466=ADVANCED_FACE('',(#3071),#2738,.F.) ;
#12467=ADVANCED_FACE('',(#3072),#12049,.F.) ;
#12468=ADVANCED_FACE('',(#3073),#2739,.F.) ;
#12469=ADVANCED_FACE('',(#3074),#12050,.F.) ;
#12470=ADVANCED_FACE('',(#3075),#2740,.F.) ;
#12471=ADVANCED_FACE('',(#3076),#12051,.F.) ;
#12472=ADVANCED_FACE('',(#3077),#2741,.F.) ;
#12473=ADVANCED_FACE('',(#3078),#12052,.F.) ;
#12474=ADVANCED_FACE('',(#3079),#2742,.F.) ;
#12475=ADVANCED_FACE('',(#3080),#12053,.F.) ;
#12476=ADVANCED_FACE('',(#3081),#2743,.F.) ;
#12477=ADVANCED_FACE('',(#3082),#12054,.F.) ;
#12478=ADVANCED_FACE('',(#3083),#2744,.F.) ;
#12479=ADVANCED_FACE('',(#3084),#12055,.F.) ;
#12480=ADVANCED_FACE('',(#3085),#2745,.F.) ;
#12481=ADVANCED_FACE('',(#3086),#12056,.F.) ;
#12482=ADVANCED_FACE('',(#3087),#2746,.F.) ;
#12483=ADVANCED_FACE('',(#3088),#12057,.F.) ;
#12484=ADVANCED_FACE('',(#3089),#2747,.F.) ;
#12485=ADVANCED_FACE('',(#3090),#12058,.F.) ;
#12486=ADVANCED_FACE('',(#3091),#2748,.F.) ;
#12487=ADVANCED_FACE('',(#3092),#12059,.F.) ;
#12488=ADVANCED_FACE('',(#3093),#2749,.F.) ;
#12489=ADVANCED_FACE('',(#3094),#2750,.F.) ;
#12490=ADVANCED_FACE('',(#3095),#2751,.F.) ;
#12491=ADVANCED_FACE('',(#3096),#2752,.F.) ;
#12492=ADVANCED_FACE('',(#3097),#2753,.F.) ;
#12493=ADVANCED_FACE('',(#3098),#2754,.F.) ;
#12494=ADVANCED_FACE('',(#3099),#2755,.F.) ;
#12495=ADVANCED_FACE('',(#3100),#2756,.F.) ;
#12496=ADVANCED_FACE('',(#3101),#2757,.F.) ;
#12497=ADVANCED_FACE('',(#3102),#2758,.F.) ;
#12498=ADVANCED_FACE('',(#3103),#2759,.F.) ;
#12499=ADVANCED_FACE('',(#3104),#2760,.F.) ;
#12500=ADVANCED_FACE('',(#3105),#2761,.F.) ;
#12501=ADVANCED_FACE('',(#3106),#2762,.F.) ;
#12502=ADVANCED_FACE('',(#3107),#2763,.F.) ;
#12503=ADVANCED_FACE('',(#3108),#2764,.F.) ;
#12504=ADVANCED_FACE('',(#3109),#2765,.F.) ;
#12505=ADVANCED_FACE('',(#3110),#2766,.F.) ;
#12506=ADVANCED_FACE('',(#3111),#2767,.F.) ;
#12507=ADVANCED_FACE('',(#3112),#2768,.F.) ;
#12508=ADVANCED_FACE('',(#3113),#2769,.F.) ;
#12509=ADVANCED_FACE('',(#3114),#2770,.F.) ;
#12510=ADVANCED_FACE('',(#3115),#2771,.F.) ;
#12511=ADVANCED_FACE('',(#3116),#2772,.F.) ;
#12512=ADVANCED_FACE('',(#3117),#2773,.F.) ;
#12513=ADVANCED_FACE('',(#3118),#2774,.F.) ;
#12514=ADVANCED_FACE('',(#3119),#2775,.F.) ;
#12515=ADVANCED_FACE('',(#3120),#2776,.F.) ;
#12516=ADVANCED_FACE('',(#3121),#2777,.T.) ;
#12517=ADVANCED_FACE('',(#3122,#759,#760,#761,#762,#763,#764,#765,#766,
#767,#768,#769,#770,#771,#772,#773,#774,#775,#776,#777,#778,#779,#780,#781,
#782,#783,#784,#785,#786,#787,#788,#789,#790,#791,#792,#793,#794,#795,#796,
#797,#798,#799,#800,#801,#802,#803,#804,#805,#806,#807,#808,#809,#810),
#12060,.T.) ;
#12518=ADVANCED_FACE('',(#3123,#811,#812,#813,#814,#815,#816,#817,#818,
#819,#820,#821,#822,#823,#824,#825,#826,#827,#828,#829,#830,#831,#832,#833,
#834,#835,#836,#837,#838),#12061,.T.) ;
#13119=CLOSED_SHELL('',(#12440,#12441,#12442,#12443,#12444,#12445,#12446,
#12447,#12448,#12449,#12450,#12451,#12452,#12453,#12454,#12455,#12456,#12457,
#12458,#12459,#12460,#12461,#12462,#12463,#12464,#12465,#12466,#12467,#12468,
#12469,#12470,#12471,#12472,#12473,#12474,#12475,#12476,#12477,#12478,#12479,
#12480,#12481,#12482,#12483,#12484,#12485,#12486,#12487,#12488,#12489,#12490,
#12491,#12492,#12493,#12494,#12495,#12496,#12497,#12498,#12499,#12500,#12501,
#12502,#12503,#12504,#12505,#12506,#12507,#12508,#12509,#12510,#12511,#12512,
#12513,#12514,#12515,#12516,#12517,#12518)) ;
#13875=AXIS2_PLACEMENT_3D('',#20264,#15924,#15925) ;
#13876=AXIS2_PLACEMENT_3D('',#20265,#15926,#15927) ;
#13877=AXIS2_PLACEMENT_3D('',#20267,#15928,#15929) ;
#13878=AXIS2_PLACEMENT_3D('',#20270,#15931,#15932) ;
#13879=AXIS2_PLACEMENT_3D('',#20271,#15933,#15934) ;
#13880=AXIS2_PLACEMENT_3D('',#20272,#15935,#15936) ;
#13881=AXIS2_PLACEMENT_3D('',#20274,#15937,#15938) ;
#13882=AXIS2_PLACEMENT_3D('',#20277,#15940,#15941) ;
#13883=AXIS2_PLACEMENT_3D('',#20278,#15942,#15943) ;
#13884=AXIS2_PLACEMENT_3D('',#20279,#15944,#15945) ;
#13885=AXIS2_PLACEMENT_3D('',#20281,#15946,#15947) ;
#13886=AXIS2_PLACEMENT_3D('',#20284,#15949,#15950) ;
#13887=AXIS2_PLACEMENT_3D('',#20285,#15951,#15952) ;
#13888=AXIS2_PLACEMENT_3D('',#20286,#15953,#15954) ;
#13889=AXIS2_PLACEMENT_3D('',#20288,#15955,#15956) ;
#13890=AXIS2_PLACEMENT_3D('',#20291,#15958,#15959) ;
#13891=AXIS2_PLACEMENT_3D('',#20292,#15960,#15961) ;
#13892=AXIS2_PLACEMENT_3D('',#20293,#15962,#15963) ;
#13893=AXIS2_PLACEMENT_3D('',#20295,#15964,#15965) ;
#13894=AXIS2_PLACEMENT_3D('',#20298,#15967,#15968) ;
#13895=AXIS2_PLACEMENT_3D('',#20299,#15969,#15970) ;
#13896=AXIS2_PLACEMENT_3D('',#20300,#15971,#15972) ;
#13897=AXIS2_PLACEMENT_3D('',#20302,#15973,#15974) ;
#13898=AXIS2_PLACEMENT_3D('',#20305,#15976,#15977) ;
#13899=AXIS2_PLACEMENT_3D('',#20306,#15978,#15979) ;
#13900=AXIS2_PLACEMENT_3D('',#20307,#15980,#15981) ;
#13901=AXIS2_PLACEMENT_3D('',#20309,#15982,#15983) ;
#13902=AXIS2_PLACEMENT_3D('',#20312,#15985,#15986) ;
#13903=AXIS2_PLACEMENT_3D('',#20313,#15987,#15988) ;
#13904=AXIS2_PLACEMENT_3D('',#20314,#15989,#15990) ;
#13905=AXIS2_PLACEMENT_3D('',#20316,#15991,#15992) ;
#13906=AXIS2_PLACEMENT_3D('',#20319,#15994,#15995) ;
#13907=AXIS2_PLACEMENT_3D('',#20320,#15996,#15997) ;
#13908=AXIS2_PLACEMENT_3D('',#20321,#15998,#15999) ;
#13909=AXIS2_PLACEMENT_3D('',#20323,#16000,#16001) ;
#13910=AXIS2_PLACEMENT_3D('',#20326,#16003,#16004) ;
#13911=AXIS2_PLACEMENT_3D('',#20327,#16005,#16006) ;
#13912=AXIS2_PLACEMENT_3D('',#20328,#16007,#16008) ;
#13913=AXIS2_PLACEMENT_3D('',#20330,#16009,#16010) ;
#13914=AXIS2_PLACEMENT_3D('',#20333,#16012,#16013) ;
#13915=AXIS2_PLACEMENT_3D('',#20334,#16014,#16015) ;
#13916=AXIS2_PLACEMENT_3D('',#20335,#16016,#16017) ;
#13917=AXIS2_PLACEMENT_3D('',#20337,#16018,#16019) ;
#13918=AXIS2_PLACEMENT_3D('',#20340,#16021,#16022) ;
#13919=AXIS2_PLACEMENT_3D('',#20341,#16023,#16024) ;
#13920=AXIS2_PLACEMENT_3D('',#20342,#16025,#16026) ;
#13921=AXIS2_PLACEMENT_3D('',#20344,#16027,#16028) ;
#13922=AXIS2_PLACEMENT_3D('',#20347,#16030,#16031) ;
#13923=AXIS2_PLACEMENT_3D('',#20348,#16032,#16033) ;
#13924=AXIS2_PLACEMENT_3D('',#20349,#16034,#16035) ;
#13925=AXIS2_PLACEMENT_3D('',#20351,#16036,#16037) ;
#13926=AXIS2_PLACEMENT_3D('',#20354,#16039,#16040) ;
#13927=AXIS2_PLACEMENT_3D('',#20355,#16041,#16042) ;
#13928=AXIS2_PLACEMENT_3D('',#20356,#16043,#16044) ;
#13929=AXIS2_PLACEMENT_3D('',#20358,#16045,#16046) ;
#13930=AXIS2_PLACEMENT_3D('',#20361,#16048,#16049) ;
#13931=AXIS2_PLACEMENT_3D('',#20362,#16050,#16051) ;
#13932=AXIS2_PLACEMENT_3D('',#20363,#16052,#16053) ;
#13933=AXIS2_PLACEMENT_3D('',#20365,#16054,#16055) ;
#13934=AXIS2_PLACEMENT_3D('',#20368,#16057,#16058) ;
#13935=AXIS2_PLACEMENT_3D('',#20369,#16059,#16060) ;
#13936=AXIS2_PLACEMENT_3D('',#20370,#16061,#16062) ;
#13937=AXIS2_PLACEMENT_3D('',#20372,#16063,#16064) ;
#13938=AXIS2_PLACEMENT_3D('',#20375,#16066,#16067) ;
#13939=AXIS2_PLACEMENT_3D('',#20376,#16068,#16069) ;
#13940=AXIS2_PLACEMENT_3D('',#20377,#16070,#16071) ;
#13941=AXIS2_PLACEMENT_3D('',#20379,#16072,#16073) ;
#13942=AXIS2_PLACEMENT_3D('',#20382,#16075,#16076) ;
#13943=AXIS2_PLACEMENT_3D('',#20383,#16077,#16078) ;
#13944=AXIS2_PLACEMENT_3D('',#20384,#16079,#16080) ;
#13945=AXIS2_PLACEMENT_3D('',#20386,#16081,#16082) ;
#13946=AXIS2_PLACEMENT_3D('',#20389,#16084,#16085) ;
#13947=AXIS2_PLACEMENT_3D('',#20390,#16086,#16087) ;
#13948=AXIS2_PLACEMENT_3D('',#20391,#16088,#16089) ;
#13949=AXIS2_PLACEMENT_3D('',#20393,#16090,#16091) ;
#13950=AXIS2_PLACEMENT_3D('',#20396,#16093,#16094) ;
#13951=AXIS2_PLACEMENT_3D('',#20397,#16095,#16096) ;
#13952=AXIS2_PLACEMENT_3D('',#20398,#16097,#16098) ;
#13953=AXIS2_PLACEMENT_3D('',#20400,#16099,#16100) ;
#13954=AXIS2_PLACEMENT_3D('',#20403,#16102,#16103) ;
#13955=AXIS2_PLACEMENT_3D('',#20404,#16104,#16105) ;
#13956=AXIS2_PLACEMENT_3D('',#20405,#16106,#16107) ;
#13957=AXIS2_PLACEMENT_3D('',#20407,#16108,#16109) ;
#13958=AXIS2_PLACEMENT_3D('',#20410,#16111,#16112) ;
#13959=AXIS2_PLACEMENT_3D('',#20411,#16113,#16114) ;
#13960=AXIS2_PLACEMENT_3D('',#20412,#16115,#16116) ;
#13961=AXIS2_PLACEMENT_3D('',#20414,#16117,#16118) ;
#13962=AXIS2_PLACEMENT_3D('',#20417,#16120,#16121) ;
#13963=AXIS2_PLACEMENT_3D('',#20418,#16122,#16123) ;
#13964=AXIS2_PLACEMENT_3D('',#20419,#16124,#16125) ;
#13965=AXIS2_PLACEMENT_3D('',#20421,#16126,#16127) ;
#13966=AXIS2_PLACEMENT_3D('',#20424,#16129,#16130) ;
#13967=AXIS2_PLACEMENT_3D('',#20425,#16131,#16132) ;
#13968=AXIS2_PLACEMENT_3D('',#20426,#16133,#16134) ;
#13969=AXIS2_PLACEMENT_3D('',#20428,#16135,#16136) ;
#13970=AXIS2_PLACEMENT_3D('',#20431,#16138,#16139) ;
#13971=AXIS2_PLACEMENT_3D('',#20432,#16140,#16141) ;
#13972=AXIS2_PLACEMENT_3D('',#20433,#16142,#16143) ;
#13973=AXIS2_PLACEMENT_3D('',#20435,#16144,#16145) ;
#13974=AXIS2_PLACEMENT_3D('',#20438,#16147,#16148) ;
#13975=AXIS2_PLACEMENT_3D('',#20439,#16149,#16150) ;
#13976=AXIS2_PLACEMENT_3D('',#20441,#16151,#16152) ;
#13977=AXIS2_PLACEMENT_3D('',#20444,#16154,#16155) ;
#13978=AXIS2_PLACEMENT_3D('',#20445,#16156,#16157) ;
#13979=AXIS2_PLACEMENT_3D('',#20447,#16158,#16159) ;
#13980=AXIS2_PLACEMENT_3D('',#20450,#16161,#16162) ;
#13981=AXIS2_PLACEMENT_3D('',#20451,#16163,#16164) ;
#13982=AXIS2_PLACEMENT_3D('',#20453,#16165,#16166) ;
#13983=AXIS2_PLACEMENT_3D('',#20456,#16168,#16169) ;
#13984=AXIS2_PLACEMENT_3D('',#20457,#16170,#16171) ;
#13985=AXIS2_PLACEMENT_3D('',#20459,#16172,#16173) ;
#13986=AXIS2_PLACEMENT_3D('',#20462,#16175,#16176) ;
#13987=AXIS2_PLACEMENT_3D('',#20463,#16177,#16178) ;
#13988=AXIS2_PLACEMENT_3D('',#20465,#16179,#16180) ;
#13989=AXIS2_PLACEMENT_3D('',#20468,#16182,#16183) ;
#13990=AXIS2_PLACEMENT_3D('',#20469,#16184,#16185) ;
#13991=AXIS2_PLACEMENT_3D('',#20471,#16186,#16187) ;
#13992=AXIS2_PLACEMENT_3D('',#20474,#16189,#16190) ;
#13993=AXIS2_PLACEMENT_3D('',#20475,#16191,#16192) ;
#13994=AXIS2_PLACEMENT_3D('',#20477,#16193,#16194) ;
#13995=AXIS2_PLACEMENT_3D('',#20480,#16196,#16197) ;
#13996=AXIS2_PLACEMENT_3D('',#20481,#16198,#16199) ;
#13997=AXIS2_PLACEMENT_3D('',#20483,#16200,#16201) ;
#13998=AXIS2_PLACEMENT_3D('',#20486,#16203,#16204) ;
#13999=AXIS2_PLACEMENT_3D('',#20487,#16205,#16206) ;
#14000=AXIS2_PLACEMENT_3D('',#20489,#16207,#16208) ;
#14001=AXIS2_PLACEMENT_3D('',#20492,#16210,#16211) ;
#14002=AXIS2_PLACEMENT_3D('',#20493,#16212,#16213) ;
#14003=AXIS2_PLACEMENT_3D('',#20495,#16214,#16215) ;
#14004=AXIS2_PLACEMENT_3D('',#20498,#16217,#16218) ;
#14005=AXIS2_PLACEMENT_3D('',#20499,#16219,#16220) ;
#14006=AXIS2_PLACEMENT_3D('',#20501,#16221,#16222) ;
#14007=AXIS2_PLACEMENT_3D('',#20504,#16224,#16225) ;
#14008=AXIS2_PLACEMENT_3D('',#20505,#16226,#16227) ;
#14009=AXIS2_PLACEMENT_3D('',#20507,#16228,#16229) ;
#14010=AXIS2_PLACEMENT_3D('',#20510,#16231,#16232) ;
#14011=AXIS2_PLACEMENT_3D('',#20511,#16233,#16234) ;
#14012=AXIS2_PLACEMENT_3D('',#20513,#16235,#16236) ;
#14013=AXIS2_PLACEMENT_3D('',#20516,#16238,#16239) ;
#14014=AXIS2_PLACEMENT_3D('',#20517,#16240,#16241) ;
#14015=AXIS2_PLACEMENT_3D('',#20519,#16242,#16243) ;
#14016=AXIS2_PLACEMENT_3D('',#20522,#16245,#16246) ;
#14017=AXIS2_PLACEMENT_3D('',#20523,#16247,#16248) ;
#14018=AXIS2_PLACEMENT_3D('',#20525,#16249,#16250) ;
#14019=AXIS2_PLACEMENT_3D('',#20528,#16252,#16253) ;
#14020=AXIS2_PLACEMENT_3D('',#20529,#16254,#16255) ;
#14021=AXIS2_PLACEMENT_3D('',#20531,#16256,#16257) ;
#14022=AXIS2_PLACEMENT_3D('',#20534,#16259,#16260) ;
#14023=AXIS2_PLACEMENT_3D('',#20535,#16261,#16262) ;
#14024=AXIS2_PLACEMENT_3D('',#20537,#16263,#16264) ;
#14025=AXIS2_PLACEMENT_3D('',#20540,#16266,#16267) ;
#14026=AXIS2_PLACEMENT_3D('',#20541,#16268,#16269) ;
#14027=AXIS2_PLACEMENT_3D('',#20543,#16270,#16271) ;
#14028=AXIS2_PLACEMENT_3D('',#20546,#16273,#16274) ;
#14029=AXIS2_PLACEMENT_3D('',#20547,#16275,#16276) ;
#14030=AXIS2_PLACEMENT_3D('',#20549,#16277,#16278) ;
#14031=AXIS2_PLACEMENT_3D('',#20552,#16280,#16281) ;
#14032=AXIS2_PLACEMENT_3D('',#20553,#16282,#16283) ;
#14033=AXIS2_PLACEMENT_3D('',#20555,#16284,#16285) ;
#14034=AXIS2_PLACEMENT_3D('',#20558,#16287,#16288) ;
#14035=AXIS2_PLACEMENT_3D('',#20559,#16289,#16290) ;
#14036=AXIS2_PLACEMENT_3D('',#20561,#16291,#16292) ;
#14037=AXIS2_PLACEMENT_3D('',#20564,#16294,#16295) ;
#14038=AXIS2_PLACEMENT_3D('',#20565,#16296,#16297) ;
#14039=AXIS2_PLACEMENT_3D('',#20567,#16298,#16299) ;
#14040=AXIS2_PLACEMENT_3D('',#20570,#16301,#16302) ;
#14041=AXIS2_PLACEMENT_3D('',#20571,#16303,#16304) ;
#14042=AXIS2_PLACEMENT_3D('',#20573,#16305,#16306) ;
#14043=AXIS2_PLACEMENT_3D('',#20576,#16308,#16309) ;
#14044=AXIS2_PLACEMENT_3D('',#20577,#16310,#16311) ;
#14045=AXIS2_PLACEMENT_3D('',#20579,#16312,#16313) ;
#14046=AXIS2_PLACEMENT_3D('',#20582,#16315,#16316) ;
#14047=AXIS2_PLACEMENT_3D('',#20583,#16317,#16318) ;
#14048=AXIS2_PLACEMENT_3D('',#20585,#16319,#16320) ;
#14049=AXIS2_PLACEMENT_3D('',#20588,#16322,#16323) ;
#14050=AXIS2_PLACEMENT_3D('',#20589,#16324,#16325) ;
#14051=AXIS2_PLACEMENT_3D('',#20591,#16326,#16327) ;
#14052=AXIS2_PLACEMENT_3D('',#20594,#16329,#16330) ;
#14053=AXIS2_PLACEMENT_3D('',#20595,#16331,#16332) ;
#14054=AXIS2_PLACEMENT_3D('',#20597,#16333,#16334) ;
#14055=AXIS2_PLACEMENT_3D('',#20600,#16336,#16337) ;
#14056=AXIS2_PLACEMENT_3D('',#20601,#16338,#16339) ;
#14057=AXIS2_PLACEMENT_3D('',#20603,#16340,#16341) ;
#14058=AXIS2_PLACEMENT_3D('',#20606,#16343,#16344) ;
#14059=AXIS2_PLACEMENT_3D('',#20607,#16345,#16346) ;
#14060=AXIS2_PLACEMENT_3D('',#20608,#16347,#16348) ;
#15924=DIRECTION('axis',(0.,0.,1.)) ;
#15925=DIRECTION('refdir',(1.,0.,0.)) ;
#15926=DIRECTION('center_axis',(0.,1.,0.)) ;
#15927=DIRECTION('ref_axis',(1.,0.,0.)) ;
#15928=DIRECTION('center_axis',(0.,1.,0.)) ;
#15929=DIRECTION('ref_axis',(1.,0.,0.)) ;
#15930=DIRECTION('',(0.,1.,0.)) ;
#15931=DIRECTION('center_axis',(0.,1.,0.)) ;
#15932=DIRECTION('ref_axis',(1.,0.,0.)) ;
#15933=DIRECTION('center_axis',(0.,1.,0.)) ;
#15934=DIRECTION('ref_axis',(1.,0.,0.)) ;
#15935=DIRECTION('center_axis',(0.,1.,0.)) ;
#15936=DIRECTION('ref_axis',(1.,0.,0.)) ;
#15937=DIRECTION('center_axis',(0.,1.,0.)) ;
#15938=DIRECTION('ref_axis',(1.,0.,0.)) ;
#15939=DIRECTION('',(0.,1.,0.)) ;
#15940=DIRECTION('center_axis',(0.,1.,0.)) ;
#15941=DIRECTION('ref_axis',(1.,0.,0.)) ;
#15942=DIRECTION('center_axis',(0.,1.,0.)) ;
#15943=DIRECTION('ref_axis',(1.,0.,0.)) ;
#15944=DIRECTION('center_axis',(0.,1.,0.)) ;
#15945=DIRECTION('ref_axis',(1.,0.,0.)) ;
#15946=DIRECTION('center_axis',(0.,1.,0.)) ;
#15947=DIRECTION('ref_axis',(1.,0.,0.)) ;
#15948=DIRECTION('',(0.,1.,0.)) ;
#15949=DIRECTION('center_axis',(0.,1.,0.)) ;
#15950=DIRECTION('ref_axis',(1.,0.,0.)) ;
#15951=DIRECTION('center_axis',(0.,1.,0.)) ;
#15952=DIRECTION('ref_axis',(1.,0.,0.)) ;
#15953=DIRECTION('center_axis',(0.,1.,0.)) ;
#15954=DIRECTION('ref_axis',(1.,0.,0.)) ;
#15955=DIRECTION('center_axis',(0.,1.,0.)) ;
#15956=DIRECTION('ref_axis',(1.,0.,0.)) ;
#15957=DIRECTION('',(0.,1.,0.)) ;
#15958=DIRECTION('center_axis',(0.,1.,0.)) ;
#15959=DIRECTION('ref_axis',(1.,0.,0.)) ;
#15960=DIRECTION('center_axis',(0.,1.,0.)) ;
#15961=DIRECTION('ref_axis',(1.,0.,0.)) ;
#15962=DIRECTION('center_axis',(0.,1.,0.)) ;
#15963=DIRECTION('ref_axis',(1.,0.,0.)) ;
#15964=DIRECTION('center_axis',(0.,1.,0.)) ;
#15965=DIRECTION('ref_axis',(1.,0.,0.)) ;
#15966=DIRECTION('',(0.,1.,0.)) ;
#15967=DIRECTION('center_axis',(0.,1.,0.)) ;
#15968=DIRECTION('ref_axis',(1.,0.,0.)) ;
#15969=DIRECTION('center_axis',(0.,1.,0.)) ;
#15970=DIRECTION('ref_axis',(1.,0.,0.)) ;
#15971=DIRECTION('center_axis',(0.,1.,0.)) ;
#15972=DIRECTION('ref_axis',(1.,0.,0.)) ;
#15973=DIRECTION('center_axis',(0.,1.,0.)) ;
#15974=DIRECTION('ref_axis',(1.,0.,0.)) ;
#15975=DIRECTION('',(0.,1.,0.)) ;
#15976=DIRECTION('center_axis',(0.,1.,0.)) ;
#15977=DIRECTION('ref_axis',(1.,0.,0.)) ;
#15978=DIRECTION('center_axis',(0.,1.,0.)) ;
#15979=DIRECTION('ref_axis',(1.,0.,0.)) ;
#15980=DIRECTION('center_axis',(0.,1.,0.)) ;
#15981=DIRECTION('ref_axis',(1.,0.,0.)) ;
#15982=DIRECTION('center_axis',(0.,1.,0.)) ;
#15983=DIRECTION('ref_axis',(1.,0.,0.)) ;
#15984=DIRECTION('',(0.,1.,0.)) ;
#15985=DIRECTION('center_axis',(0.,1.,0.)) ;
#15986=DIRECTION('ref_axis',(1.,0.,0.)) ;
#15987=DIRECTION('center_axis',(0.,1.,0.)) ;
#15988=DIRECTION('ref_axis',(1.,0.,0.)) ;
#15989=DIRECTION('center_axis',(0.,1.,0.)) ;
#15990=DIRECTION('ref_axis',(1.,0.,0.)) ;
#15991=DIRECTION('center_axis',(0.,1.,0.)) ;
#15992=DIRECTION('ref_axis',(1.,0.,0.)) ;
#15993=DIRECTION('',(0.,1.,0.)) ;
#15994=DIRECTION('center_axis',(0.,1.,0.)) ;
#15995=DIRECTION('ref_axis',(1.,0.,0.)) ;
#15996=DIRECTION('center_axis',(0.,1.,0.)) ;
#15997=DIRECTION('ref_axis',(1.,0.,0.)) ;
#15998=DIRECTION('center_axis',(0.,1.,0.)) ;
#15999=DIRECTION('ref_axis',(1.,0.,0.)) ;
#16000=DIRECTION('center_axis',(0.,1.,0.)) ;
#16001=DIRECTION('ref_axis',(1.,0.,0.)) ;
#16002=DIRECTION('',(0.,1.,0.)) ;
#16003=DIRECTION('center_axis',(0.,1.,0.)) ;
#16004=DIRECTION('ref_axis',(1.,0.,0.)) ;
#16005=DIRECTION('center_axis',(0.,1.,0.)) ;
#16006=DIRECTION('ref_axis',(1.,0.,0.)) ;
#16007=DIRECTION('center_axis',(0.,1.,0.)) ;
#16008=DIRECTION('ref_axis',(1.,0.,0.)) ;
#16009=DIRECTION('center_axis',(0.,1.,0.)) ;
#16010=DIRECTION('ref_axis',(1.,0.,0.)) ;
#16011=DIRECTION('',(0.,1.,0.)) ;
#16012=DIRECTION('center_axis',(0.,1.,0.)) ;
#16013=DIRECTION('ref_axis',(1.,0.,0.)) ;
#16014=DIRECTION('center_axis',(0.,1.,0.)) ;
#16015=DIRECTION('ref_axis',(1.,0.,0.)) ;
#16016=DIRECTION('center_axis',(0.,1.,0.)) ;
#16017=DIRECTION('ref_axis',(1.,0.,0.)) ;
#16018=DIRECTION('center_axis',(0.,1.,0.)) ;
#16019=DIRECTION('ref_axis',(1.,0.,0.)) ;
#16020=DIRECTION('',(0.,1.,0.)) ;
#16021=DIRECTION('center_axis',(0.,1.,0.)) ;
#16022=DIRECTION('ref_axis',(1.,0.,0.)) ;
#16023=DIRECTION('center_axis',(0.,1.,0.)) ;
#16024=DIRECTION('ref_axis',(1.,0.,0.)) ;
#16025=DIRECTION('center_axis',(0.,1.,0.)) ;
#16026=DIRECTION('ref_axis',(1.,0.,0.)) ;
#16027=DIRECTION('center_axis',(0.,1.,0.)) ;
#16028=DIRECTION('ref_axis',(1.,0.,0.)) ;
#16029=DIRECTION('',(0.,1.,0.)) ;
#16030=DIRECTION('center_axis',(0.,1.,0.)) ;
#16031=DIRECTION('ref_axis',(1.,0.,0.)) ;
#16032=DIRECTION('center_axis',(0.,1.,0.)) ;
#16033=DIRECTION('ref_axis',(1.,0.,0.)) ;
#16034=DIRECTION('center_axis',(0.,1.,0.)) ;
#16035=DIRECTION('ref_axis',(1.,0.,0.)) ;
#16036=DIRECTION('center_axis',(0.,1.,0.)) ;
#16037=DIRECTION('ref_axis',(1.,0.,0.)) ;
#16038=DIRECTION('',(0.,1.,0.)) ;
#16039=DIRECTION('center_axis',(0.,1.,0.)) ;
#16040=DIRECTION('ref_axis',(1.,0.,0.)) ;
#16041=DIRECTION('center_axis',(0.,1.,0.)) ;
#16042=DIRECTION('ref_axis',(1.,0.,0.)) ;
#16043=DIRECTION('center_axis',(0.,1.,0.)) ;
#16044=DIRECTION('ref_axis',(1.,0.,0.)) ;
#16045=DIRECTION('center_axis',(0.,1.,0.)) ;
#16046=DIRECTION('ref_axis',(1.,0.,0.)) ;
#16047=DIRECTION('',(0.,1.,0.)) ;
#16048=DIRECTION('center_axis',(0.,1.,0.)) ;
#16049=DIRECTION('ref_axis',(1.,0.,0.)) ;
#16050=DIRECTION('center_axis',(0.,1.,0.)) ;
#16051=DIRECTION('ref_axis',(1.,0.,0.)) ;
#16052=DIRECTION('center_axis',(0.,1.,0.)) ;
#16053=DIRECTION('ref_axis',(1.,0.,0.)) ;
#16054=DIRECTION('center_axis',(0.,1.,0.)) ;
#16055=DIRECTION('ref_axis',(1.,0.,0.)) ;
#16056=DIRECTION('',(0.,1.,0.)) ;
#16057=DIRECTION('center_axis',(0.,1.,0.)) ;
#16058=DIRECTION('ref_axis',(1.,0.,0.)) ;
#16059=DIRECTION('center_axis',(0.,1.,0.)) ;
#16060=DIRECTION('ref_axis',(1.,0.,0.)) ;
#16061=DIRECTION('center_axis',(0.,1.,0.)) ;
#16062=DIRECTION('ref_axis',(1.,0.,0.)) ;
#16063=DIRECTION('center_axis',(0.,1.,0.)) ;
#16064=DIRECTION('ref_axis',(1.,0.,0.)) ;
#16065=DIRECTION('',(0.,1.,0.)) ;
#16066=DIRECTION('center_axis',(0.,1.,0.)) ;
#16067=DIRECTION('ref_axis',(1.,0.,0.)) ;
#16068=DIRECTION('center_axis',(0.,1.,0.)) ;
#16069=DIRECTION('ref_axis',(1.,0.,0.)) ;
#16070=DIRECTION('center_axis',(0.,1.,0.)) ;
#16071=DIRECTION('ref_axis',(1.,0.,0.)) ;
#16072=DIRECTION('center_axis',(0.,1.,0.)) ;
#16073=DIRECTION('ref_axis',(1.,0.,0.)) ;
#16074=DIRECTION('',(0.,1.,0.)) ;
#16075=DIRECTION('center_axis',(0.,1.,0.)) ;
#16076=DIRECTION('ref_axis',(1.,0.,0.)) ;
#16077=DIRECTION('center_axis',(0.,1.,0.)) ;
#16078=DIRECTION('ref_axis',(1.,0.,0.)) ;
#16079=DIRECTION('center_axis',(0.,1.,0.)) ;
#16080=DIRECTION('ref_axis',(1.,0.,0.)) ;
#16081=DIRECTION('center_axis',(0.,1.,0.)) ;
#16082=DIRECTION('ref_axis',(1.,0.,0.)) ;
#16083=DIRECTION('',(0.,1.,0.)) ;
#16084=DIRECTION('center_axis',(0.,1.,0.)) ;
#16085=DIRECTION('ref_axis',(1.,0.,0.)) ;
#16086=DIRECTION('center_axis',(0.,1.,0.)) ;
#16087=DIRECTION('ref_axis',(1.,0.,0.)) ;
#16088=DIRECTION('center_axis',(0.,1.,0.)) ;
#16089=DIRECTION('ref_axis',(1.,0.,0.)) ;
#16090=DIRECTION('center_axis',(0.,1.,0.)) ;
#16091=DIRECTION('ref_axis',(1.,0.,0.)) ;
#16092=DIRECTION('',(0.,1.,0.)) ;
#16093=DIRECTION('center_axis',(0.,1.,0.)) ;
#16094=DIRECTION('ref_axis',(1.,0.,0.)) ;
#16095=DIRECTION('center_axis',(0.,1.,0.)) ;
#16096=DIRECTION('ref_axis',(1.,0.,0.)) ;
#16097=DIRECTION('center_axis',(0.,1.,0.)) ;
#16098=DIRECTION('ref_axis',(1.,0.,0.)) ;
#16099=DIRECTION('center_axis',(0.,1.,0.)) ;
#16100=DIRECTION('ref_axis',(1.,0.,0.)) ;
#16101=DIRECTION('',(0.,1.,0.)) ;
#16102=DIRECTION('center_axis',(0.,1.,0.)) ;
#16103=DIRECTION('ref_axis',(1.,0.,0.)) ;
#16104=DIRECTION('center_axis',(0.,1.,0.)) ;
#16105=DIRECTION('ref_axis',(1.,0.,0.)) ;
#16106=DIRECTION('center_axis',(0.,1.,0.)) ;
#16107=DIRECTION('ref_axis',(1.,0.,0.)) ;
#16108=DIRECTION('center_axis',(0.,1.,0.)) ;
#16109=DIRECTION('ref_axis',(1.,0.,0.)) ;
#16110=DIRECTION('',(0.,1.,0.)) ;
#16111=DIRECTION('center_axis',(0.,1.,0.)) ;
#16112=DIRECTION('ref_axis',(1.,0.,0.)) ;
#16113=DIRECTION('center_axis',(0.,1.,0.)) ;
#16114=DIRECTION('ref_axis',(1.,0.,0.)) ;
#16115=DIRECTION('center_axis',(0.,1.,0.)) ;
#16116=DIRECTION('ref_axis',(1.,0.,0.)) ;
#16117=DIRECTION('center_axis',(0.,1.,0.)) ;
#16118=DIRECTION('ref_axis',(1.,0.,0.)) ;
#16119=DIRECTION('',(0.,1.,0.)) ;
#16120=DIRECTION('center_axis',(0.,1.,0.)) ;
#16121=DIRECTION('ref_axis',(1.,0.,0.)) ;
#16122=DIRECTION('center_axis',(0.,1.,0.)) ;
#16123=DIRECTION('ref_axis',(1.,0.,0.)) ;
#16124=DIRECTION('center_axis',(0.,1.,0.)) ;
#16125=DIRECTION('ref_axis',(1.,0.,0.)) ;
#16126=DIRECTION('center_axis',(0.,1.,0.)) ;
#16127=DIRECTION('ref_axis',(1.,0.,0.)) ;
#16128=DIRECTION('',(0.,1.,0.)) ;
#16129=DIRECTION('center_axis',(0.,1.,0.)) ;
#16130=DIRECTION('ref_axis',(1.,0.,0.)) ;
#16131=DIRECTION('center_axis',(0.,1.,0.)) ;
#16132=DIRECTION('ref_axis',(1.,0.,0.)) ;
#16133=DIRECTION('center_axis',(0.,1.,0.)) ;
#16134=DIRECTION('ref_axis',(1.,0.,0.)) ;
#16135=DIRECTION('center_axis',(0.,1.,0.)) ;
#16136=DIRECTION('ref_axis',(1.,0.,0.)) ;
#16137=DIRECTION('',(0.,1.,0.)) ;
#16138=DIRECTION('center_axis',(0.,1.,0.)) ;
#16139=DIRECTION('ref_axis',(1.,0.,0.)) ;
#16140=DIRECTION('center_axis',(0.,1.,0.)) ;
#16141=DIRECTION('ref_axis',(1.,0.,0.)) ;
#16142=DIRECTION('center_axis',(0.,1.,0.)) ;
#16143=DIRECTION('ref_axis',(1.,0.,0.)) ;
#16144=DIRECTION('center_axis',(0.,1.,0.)) ;
#16145=DIRECTION('ref_axis',(1.,0.,0.)) ;
#16146=DIRECTION('',(0.,1.,0.)) ;
#16147=DIRECTION('center_axis',(0.,-1.,0.)) ;
#16148=DIRECTION('ref_axis',(1.,0.,0.)) ;
#16149=DIRECTION('center_axis',(0.,1.,0.)) ;
#16150=DIRECTION('ref_axis',(1.,0.,0.)) ;
#16151=DIRECTION('center_axis',(0.,1.,0.)) ;
#16152=DIRECTION('ref_axis',(1.,0.,0.)) ;
#16153=DIRECTION('',(0.,1.,0.)) ;
#16154=DIRECTION('center_axis',(0.,-1.,0.)) ;
#16155=DIRECTION('ref_axis',(1.,0.,0.)) ;
#16156=DIRECTION('center_axis',(0.,1.,0.)) ;
#16157=DIRECTION('ref_axis',(1.,0.,0.)) ;
#16158=DIRECTION('center_axis',(0.,1.,0.)) ;
#16159=DIRECTION('ref_axis',(1.,0.,0.)) ;
#16160=DIRECTION('',(0.,1.,0.)) ;
#16161=DIRECTION('center_axis',(0.,-1.,0.)) ;
#16162=DIRECTION('ref_axis',(1.,0.,0.)) ;
#16163=DIRECTION('center_axis',(0.,1.,0.)) ;
#16164=DIRECTION('ref_axis',(1.,0.,0.)) ;
#16165=DIRECTION('center_axis',(0.,1.,0.)) ;
#16166=DIRECTION('ref_axis',(1.,0.,0.)) ;
#16167=DIRECTION('',(0.,1.,0.)) ;
#16168=DIRECTION('center_axis',(0.,-1.,0.)) ;
#16169=DIRECTION('ref_axis',(1.,0.,0.)) ;
#16170=DIRECTION('center_axis',(0.,1.,0.)) ;
#16171=DIRECTION('ref_axis',(1.,0.,0.)) ;
#16172=DIRECTION('center_axis',(0.,1.,0.)) ;
#16173=DIRECTION('ref_axis',(1.,0.,0.)) ;
#16174=DIRECTION('',(0.,1.,0.)) ;
#16175=DIRECTION('center_axis',(0.,-1.,0.)) ;
#16176=DIRECTION('ref_axis',(1.,0.,0.)) ;
#16177=DIRECTION('center_axis',(0.,1.,0.)) ;
#16178=DIRECTION('ref_axis',(1.,0.,0.)) ;
#16179=DIRECTION('center_axis',(0.,1.,0.)) ;
#16180=DIRECTION('ref_axis',(1.,0.,0.)) ;
#16181=DIRECTION('',(0.,1.,0.)) ;
#16182=DIRECTION('center_axis',(0.,-1.,0.)) ;
#16183=DIRECTION('ref_axis',(1.,0.,0.)) ;
#16184=DIRECTION('center_axis',(0.,1.,0.)) ;
#16185=DIRECTION('ref_axis',(1.,0.,0.)) ;
#16186=DIRECTION('center_axis',(0.,1.,0.)) ;
#16187=DIRECTION('ref_axis',(1.,0.,0.)) ;
#16188=DIRECTION('',(0.,1.,0.)) ;
#16189=DIRECTION('center_axis',(0.,-1.,0.)) ;
#16190=DIRECTION('ref_axis',(1.,0.,0.)) ;
#16191=DIRECTION('center_axis',(0.,1.,0.)) ;
#16192=DIRECTION('ref_axis',(1.,0.,0.)) ;
#16193=DIRECTION('center_axis',(0.,1.,0.)) ;
#16194=DIRECTION('ref_axis',(1.,0.,0.)) ;
#16195=DIRECTION('',(0.,1.,0.)) ;
#16196=DIRECTION('center_axis',(0.,-1.,0.)) ;
#16197=DIRECTION('ref_axis',(1.,0.,0.)) ;
#16198=DIRECTION('center_axis',(0.,1.,0.)) ;
#16199=DIRECTION('ref_axis',(1.,0.,0.)) ;
#16200=DIRECTION('center_axis',(0.,1.,0.)) ;
#16201=DIRECTION('ref_axis',(1.,0.,0.)) ;
#16202=DIRECTION('',(0.,1.,0.)) ;
#16203=DIRECTION('center_axis',(0.,-1.,0.)) ;
#16204=DIRECTION('ref_axis',(1.,0.,0.)) ;
#16205=DIRECTION('center_axis',(0.,1.,0.)) ;
#16206=DIRECTION('ref_axis',(1.,0.,0.)) ;
#16207=DIRECTION('center_axis',(0.,1.,0.)) ;
#16208=DIRECTION('ref_axis',(1.,0.,0.)) ;
#16209=DIRECTION('',(0.,1.,0.)) ;
#16210=DIRECTION('center_axis',(0.,-1.,0.)) ;
#16211=DIRECTION('ref_axis',(1.,0.,0.)) ;
#16212=DIRECTION('center_axis',(0.,1.,0.)) ;
#16213=DIRECTION('ref_axis',(1.,0.,0.)) ;
#16214=DIRECTION('center_axis',(0.,1.,0.)) ;
#16215=DIRECTION('ref_axis',(1.,0.,0.)) ;
#16216=DIRECTION('',(0.,1.,0.)) ;
#16217=DIRECTION('center_axis',(0.,-1.,0.)) ;
#16218=DIRECTION('ref_axis',(1.,0.,0.)) ;
#16219=DIRECTION('center_axis',(0.,1.,0.)) ;
#16220=DIRECTION('ref_axis',(1.,0.,0.)) ;
#16221=DIRECTION('center_axis',(0.,1.,0.)) ;
#16222=DIRECTION('ref_axis',(1.,0.,0.)) ;
#16223=DIRECTION('',(0.,1.,0.)) ;
#16224=DIRECTION('center_axis',(0.,-1.,0.)) ;
#16225=DIRECTION('ref_axis',(1.,0.,0.)) ;
#16226=DIRECTION('center_axis',(0.,1.,0.)) ;
#16227=DIRECTION('ref_axis',(1.,0.,0.)) ;
#16228=DIRECTION('center_axis',(0.,1.,0.)) ;
#16229=DIRECTION('ref_axis',(1.,0.,0.)) ;
#16230=DIRECTION('',(0.,1.,0.)) ;
#16231=DIRECTION('center_axis',(0.,-1.,0.)) ;
#16232=DIRECTION('ref_axis',(1.,0.,0.)) ;
#16233=DIRECTION('center_axis',(0.,1.,0.)) ;
#16234=DIRECTION('ref_axis',(1.,0.,0.)) ;
#16235=DIRECTION('center_axis',(0.,1.,0.)) ;
#16236=DIRECTION('ref_axis',(1.,0.,0.)) ;
#16237=DIRECTION('',(0.,1.,0.)) ;
#16238=DIRECTION('center_axis',(0.,-1.,0.)) ;
#16239=DIRECTION('ref_axis',(1.,0.,0.)) ;
#16240=DIRECTION('center_axis',(0.,1.,0.)) ;
#16241=DIRECTION('ref_axis',(1.,0.,0.)) ;
#16242=DIRECTION('center_axis',(0.,1.,0.)) ;
#16243=DIRECTION('ref_axis',(1.,0.,0.)) ;
#16244=DIRECTION('',(0.,1.,0.)) ;
#16245=DIRECTION('center_axis',(0.,-1.,0.)) ;
#16246=DIRECTION('ref_axis',(1.,0.,0.)) ;
#16247=DIRECTION('center_axis',(0.,1.,0.)) ;
#16248=DIRECTION('ref_axis',(1.,0.,0.)) ;
#16249=DIRECTION('center_axis',(0.,1.,0.)) ;
#16250=DIRECTION('ref_axis',(1.,0.,0.)) ;
#16251=DIRECTION('',(0.,1.,0.)) ;
#16252=DIRECTION('center_axis',(0.,-1.,0.)) ;
#16253=DIRECTION('ref_axis',(1.,0.,0.)) ;
#16254=DIRECTION('center_axis',(0.,1.,0.)) ;
#16255=DIRECTION('ref_axis',(1.,0.,0.)) ;
#16256=DIRECTION('center_axis',(0.,1.,0.)) ;
#16257=DIRECTION('ref_axis',(1.,0.,0.)) ;
#16258=DIRECTION('',(0.,1.,0.)) ;
#16259=DIRECTION('center_axis',(0.,-1.,0.)) ;
#16260=DIRECTION('ref_axis',(1.,0.,0.)) ;
#16261=DIRECTION('center_axis',(0.,1.,0.)) ;
#16262=DIRECTION('ref_axis',(1.,0.,0.)) ;
#16263=DIRECTION('center_axis',(0.,1.,0.)) ;
#16264=DIRECTION('ref_axis',(1.,0.,0.)) ;
#16265=DIRECTION('',(0.,1.,0.)) ;
#16266=DIRECTION('center_axis',(0.,-1.,0.)) ;
#16267=DIRECTION('ref_axis',(1.,0.,0.)) ;
#16268=DIRECTION('center_axis',(0.,1.,0.)) ;
#16269=DIRECTION('ref_axis',(1.,0.,0.)) ;
#16270=DIRECTION('center_axis',(0.,1.,0.)) ;
#16271=DIRECTION('ref_axis',(1.,0.,0.)) ;
#16272=DIRECTION('',(0.,1.,0.)) ;
#16273=DIRECTION('center_axis',(0.,-1.,0.)) ;
#16274=DIRECTION('ref_axis',(1.,0.,0.)) ;
#16275=DIRECTION('center_axis',(0.,1.,0.)) ;
#16276=DIRECTION('ref_axis',(1.,0.,0.)) ;
#16277=DIRECTION('center_axis',(0.,1.,0.)) ;
#16278=DIRECTION('ref_axis',(1.,0.,0.)) ;
#16279=DIRECTION('',(0.,1.,0.)) ;
#16280=DIRECTION('center_axis',(0.,-1.,0.)) ;
#16281=DIRECTION('ref_axis',(1.,0.,0.)) ;
#16282=DIRECTION('center_axis',(0.,1.,0.)) ;
#16283=DIRECTION('ref_axis',(1.,0.,0.)) ;
#16284=DIRECTION('center_axis',(0.,1.,0.)) ;
#16285=DIRECTION('ref_axis',(1.,0.,0.)) ;
#16286=DIRECTION('',(0.,1.,0.)) ;
#16287=DIRECTION('center_axis',(0.,-1.,0.)) ;
#16288=DIRECTION('ref_axis',(1.,0.,0.)) ;
#16289=DIRECTION('center_axis',(0.,1.,0.)) ;
#16290=DIRECTION('ref_axis',(1.,0.,0.)) ;
#16291=DIRECTION('center_axis',(0.,1.,0.)) ;
#16292=DIRECTION('ref_axis',(1.,0.,0.)) ;
#16293=DIRECTION('',(0.,1.,0.)) ;
#16294=DIRECTION('center_axis',(0.,-1.,0.)) ;
#16295=DIRECTION('ref_axis',(1.,0.,0.)) ;
#16296=DIRECTION('center_axis',(0.,1.,0.)) ;
#16297=DIRECTION('ref_axis',(1.,0.,0.)) ;
#16298=DIRECTION('center_axis',(0.,1.,0.)) ;
#16299=DIRECTION('ref_axis',(1.,0.,0.)) ;
#16300=DIRECTION('',(0.,1.,0.)) ;
#16301=DIRECTION('center_axis',(0.,-1.,0.)) ;
#16302=DIRECTION('ref_axis',(1.,0.,0.)) ;
#16303=DIRECTION('center_axis',(0.,1.,0.)) ;
#16304=DIRECTION('ref_axis',(1.,0.,0.)) ;
#16305=DIRECTION('center_axis',(0.,1.,0.)) ;
#16306=DIRECTION('ref_axis',(1.,0.,0.)) ;
#16307=DIRECTION('',(0.,1.,0.)) ;
#16308=DIRECTION('center_axis',(0.,-1.,0.)) ;
#16309=DIRECTION('ref_axis',(1.,0.,0.)) ;
#16310=DIRECTION('center_axis',(0.,1.,0.)) ;
#16311=DIRECTION('ref_axis',(1.,0.,0.)) ;
#16312=DIRECTION('center_axis',(0.,1.,0.)) ;
#16313=DIRECTION('ref_axis',(1.,0.,0.)) ;
#16314=DIRECTION('',(0.,1.,0.)) ;
#16315=DIRECTION('center_axis',(0.,-1.,0.)) ;
#16316=DIRECTION('ref_axis',(1.,0.,0.)) ;
#16317=DIRECTION('center_axis',(0.,1.,0.)) ;
#16318=DIRECTION('ref_axis',(1.,0.,0.)) ;
#16319=DIRECTION('center_axis',(0.,1.,0.)) ;
#16320=DIRECTION('ref_axis',(1.,0.,0.)) ;
#16321=DIRECTION('',(0.,1.,0.)) ;
#16322=DIRECTION('center_axis',(0.,-1.,0.)) ;
#16323=DIRECTION('ref_axis',(1.,0.,0.)) ;
#16324=DIRECTION('center_axis',(0.,1.,0.)) ;
#16325=DIRECTION('ref_axis',(1.,0.,0.)) ;
#16326=DIRECTION('center_axis',(0.,1.,0.)) ;
#16327=DIRECTION('ref_axis',(1.,0.,0.)) ;
#16328=DIRECTION('',(0.,1.,0.)) ;
#16329=DIRECTION('center_axis',(0.,-1.,0.)) ;
#16330=DIRECTION('ref_axis',(1.,0.,0.)) ;
#16331=DIRECTION('center_axis',(0.,1.,0.)) ;
#16332=DIRECTION('ref_axis',(1.,0.,0.)) ;
#16333=DIRECTION('center_axis',(0.,1.,0.)) ;
#16334=DIRECTION('ref_axis',(1.,0.,0.)) ;
#16335=DIRECTION('',(0.,1.,0.)) ;
#16336=DIRECTION('center_axis',(0.,-1.,0.)) ;
#16337=DIRECTION('ref_axis',(1.,0.,0.)) ;
#16338=DIRECTION('center_axis',(0.,1.,0.)) ;
#16339=DIRECTION('ref_axis',(1.,0.,0.)) ;
#16340=DIRECTION('center_axis',(0.,1.,0.)) ;
#16341=DIRECTION('ref_axis',(1.,0.,0.)) ;
#16342=DIRECTION('',(0.,-1.,0.)) ;
#16343=DIRECTION('center_axis',(0.,-1.,0.)) ;
#16344=DIRECTION('ref_axis',(1.,0.,0.)) ;
#16345=DIRECTION('center_axis',(0.,-1.,0.)) ;
#16346=DIRECTION('ref_axis',(-1.,0.,0.)) ;
#16347=DIRECTION('center_axis',(0.,1.,0.)) ;
#16348=DIRECTION('ref_axis',(1.,0.,0.)) ;
#20264=CARTESIAN_POINT('',(0.,0.,0.)) ;
#20265=CARTESIAN_POINT('Origin',(8.72471478008953,-0.95,-1.14863049153645)) ;
#20266=CARTESIAN_POINT('',(8.57471478008953,-1.,-1.14863049153645)) ;
#20267=CARTESIAN_POINT('Origin',(8.72471478008953,-1.,-1.14863049153645)) ;
#20268=CARTESIAN_POINT('',(8.57471478008953,-0.8,-1.14863049153645)) ;
#20269=CARTESIAN_POINT('',(8.57471478008953,-0.95,-1.14863049153645)) ;
#20270=CARTESIAN_POINT('Origin',(8.72471478008953,-0.8,-1.14863049153645)) ;
#20271=CARTESIAN_POINT('Origin',(8.72471478008953,-0.8,-1.14863049153645)) ;
#20272=CARTESIAN_POINT('Origin',(8.13013988609933,-0.95,-3.36761420481279)) ;
#20273=CARTESIAN_POINT('',(7.98013988609932,-1.,-3.36761420481279)) ;
#20274=CARTESIAN_POINT('Origin',(8.13013988609933,-1.,-3.36761420481279)) ;
#20275=CARTESIAN_POINT('',(7.98013988609932,-0.8,-3.36761420481279)) ;
#20276=CARTESIAN_POINT('',(7.98013988609932,-0.95,-3.36761420481279)) ;
#20277=CARTESIAN_POINT('Origin',(8.13013988609933,-0.8,-3.36761420481279)) ;
#20278=CARTESIAN_POINT('Origin',(8.13013988609933,-0.8,-3.36761420481279)) ;
#20279=CARTESIAN_POINT('Origin',(6.98150939456287,-0.95,-5.35710057527674)) ;
#20280=CARTESIAN_POINT('',(6.83150939456287,-1.,-5.35710057527674)) ;
#20281=CARTESIAN_POINT('Origin',(6.98150939456287,-1.,-5.35710057527674)) ;
#20282=CARTESIAN_POINT('',(6.83150939456287,-0.8,-5.35710057527674)) ;
#20283=CARTESIAN_POINT('',(6.83150939456287,-0.95,-5.35710057527674)) ;
#20284=CARTESIAN_POINT('Origin',(6.98150939456287,-0.8,-5.35710057527674)) ;
#20285=CARTESIAN_POINT('Origin',(6.98150939456287,-0.8,-5.35710057527674)) ;
#20286=CARTESIAN_POINT('Origin',(5.35710057527674,-0.95,-6.98150939456287)) ;
#20287=CARTESIAN_POINT('',(5.20710057527674,-1.,-6.98150939456287)) ;
#20288=CARTESIAN_POINT('Origin',(5.35710057527674,-1.,-6.98150939456287)) ;
#20289=CARTESIAN_POINT('',(5.20710057527674,-0.8,-6.98150939456287)) ;
#20290=CARTESIAN_POINT('',(5.20710057527674,-0.95,-6.98150939456287)) ;
#20291=CARTESIAN_POINT('Origin',(5.35710057527674,-0.8,-6.98150939456287)) ;
#20292=CARTESIAN_POINT('Origin',(5.35710057527674,-0.8,-6.98150939456287)) ;
#20293=CARTESIAN_POINT('Origin',(3.36761420481279,-0.95,-8.13013988609932)) ;
#20294=CARTESIAN_POINT('',(3.21761420481279,-1.,-8.13013988609932)) ;
#20295=CARTESIAN_POINT('Origin',(3.36761420481279,-1.,-8.13013988609932)) ;
#20296=CARTESIAN_POINT('',(3.21761420481279,-0.8,-8.13013988609932)) ;
#20297=CARTESIAN_POINT('',(3.21761420481279,-0.95,-8.13013988609932)) ;
#20298=CARTESIAN_POINT('Origin',(3.36761420481279,-0.8,-8.13013988609932)) ;
#20299=CARTESIAN_POINT('Origin',(3.36761420481279,-0.8,-8.13013988609932)) ;
#20300=CARTESIAN_POINT('Origin',(1.14863049153645,-0.95,-8.72471478008953)) ;
#20301=CARTESIAN_POINT('',(0.998630491536451,-1.,-8.72471478008953)) ;
#20302=CARTESIAN_POINT('Origin',(1.14863049153645,-1.,-8.72471478008953)) ;
#20303=CARTESIAN_POINT('',(0.998630491536451,-0.8,-8.72471478008953)) ;
#20304=CARTESIAN_POINT('',(0.998630491536451,-0.95,-8.72471478008953)) ;
#20305=CARTESIAN_POINT('Origin',(1.14863049153645,-0.8,-8.72471478008953)) ;
#20306=CARTESIAN_POINT('Origin',(1.14863049153645,-0.8,-8.72471478008953)) ;
#20307=CARTESIAN_POINT('Origin',(-1.14863049153645,-0.95,-8.72471478008953)) ;
#20308=CARTESIAN_POINT('',(-1.29863049153645,-1.,-8.72471478008953)) ;
#20309=CARTESIAN_POINT('Origin',(-1.14863049153645,-1.,-8.72471478008953)) ;
#20310=CARTESIAN_POINT('',(-1.29863049153645,-0.8,-8.72471478008953)) ;
#20311=CARTESIAN_POINT('',(-1.29863049153645,-0.95,-8.72471478008953)) ;
#20312=CARTESIAN_POINT('Origin',(-1.14863049153645,-0.8,-8.72471478008953)) ;
#20313=CARTESIAN_POINT('Origin',(-1.14863049153645,-0.8,-8.72471478008953)) ;
#20314=CARTESIAN_POINT('Origin',(-3.36761420481279,-0.95,-8.13013988609933)) ;
#20315=CARTESIAN_POINT('',(-3.51761420481279,-1.,-8.13013988609933)) ;
#20316=CARTESIAN_POINT('Origin',(-3.36761420481279,-1.,-8.13013988609933)) ;
#20317=CARTESIAN_POINT('',(-3.51761420481279,-0.8,-8.13013988609933)) ;
#20318=CARTESIAN_POINT('',(-3.51761420481279,-0.95,-8.13013988609933)) ;
#20319=CARTESIAN_POINT('Origin',(-3.36761420481279,-0.8,-8.13013988609933)) ;
#20320=CARTESIAN_POINT('Origin',(-3.36761420481279,-0.8,-8.13013988609933)) ;
#20321=CARTESIAN_POINT('Origin',(-5.35710057527674,-0.95,-6.98150939456287)) ;
#20322=CARTESIAN_POINT('',(-5.50710057527674,-1.,-6.98150939456287)) ;
#20323=CARTESIAN_POINT('Origin',(-5.35710057527674,-1.,-6.98150939456287)) ;
#20324=CARTESIAN_POINT('',(-5.50710057527674,-0.8,-6.98150939456287)) ;
#20325=CARTESIAN_POINT('',(-5.50710057527674,-0.95,-6.98150939456287)) ;
#20326=CARTESIAN_POINT('Origin',(-5.35710057527674,-0.8,-6.98150939456287)) ;
#20327=CARTESIAN_POINT('Origin',(-5.35710057527674,-0.8,-6.98150939456287)) ;
#20328=CARTESIAN_POINT('Origin',(-6.98150939456287,-0.95,-5.35710057527674)) ;
#20329=CARTESIAN_POINT('',(-7.13150939456287,-1.,-5.35710057527674)) ;
#20330=CARTESIAN_POINT('Origin',(-6.98150939456287,-1.,-5.35710057527674)) ;
#20331=CARTESIAN_POINT('',(-7.13150939456287,-0.8,-5.35710057527674)) ;
#20332=CARTESIAN_POINT('',(-7.13150939456287,-0.95,-5.35710057527674)) ;
#20333=CARTESIAN_POINT('Origin',(-6.98150939456287,-0.8,-5.35710057527674)) ;
#20334=CARTESIAN_POINT('Origin',(-6.98150939456287,-0.8,-5.35710057527674)) ;
#20335=CARTESIAN_POINT('Origin',(-8.13013988609933,-0.95,-3.36761420481279)) ;
#20336=CARTESIAN_POINT('',(-8.28013988609933,-1.,-3.36761420481279)) ;
#20337=CARTESIAN_POINT('Origin',(-8.13013988609933,-1.,-3.36761420481279)) ;
#20338=CARTESIAN_POINT('',(-8.28013988609933,-0.8,-3.36761420481279)) ;
#20339=CARTESIAN_POINT('',(-8.28013988609933,-0.95,-3.36761420481279)) ;
#20340=CARTESIAN_POINT('Origin',(-8.13013988609933,-0.8,-3.36761420481279)) ;
#20341=CARTESIAN_POINT('Origin',(-8.13013988609933,-0.8,-3.36761420481279)) ;
#20342=CARTESIAN_POINT('Origin',(-8.72471478008953,-0.95,-1.14863049153645)) ;
#20343=CARTESIAN_POINT('',(-8.87471478008953,-1.,-1.14863049153645)) ;
#20344=CARTESIAN_POINT('Origin',(-8.72471478008953,-1.,-1.14863049153645)) ;
#20345=CARTESIAN_POINT('',(-8.87471478008953,-0.8,-1.14863049153645)) ;
#20346=CARTESIAN_POINT('',(-8.87471478008953,-0.95,-1.14863049153645)) ;
#20347=CARTESIAN_POINT('Origin',(-8.72471478008953,-0.8,-1.14863049153645)) ;
#20348=CARTESIAN_POINT('Origin',(-8.72471478008953,-0.8,-1.14863049153645)) ;
#20349=CARTESIAN_POINT('Origin',(-8.72471478008953,-0.95,1.14863049153645)) ;
#20350=CARTESIAN_POINT('',(-8.87471478008953,-1.,1.14863049153645)) ;
#20351=CARTESIAN_POINT('Origin',(-8.72471478008953,-1.,1.14863049153645)) ;
#20352=CARTESIAN_POINT('',(-8.87471478008953,-0.8,1.14863049153645)) ;
#20353=CARTESIAN_POINT('',(-8.87471478008953,-0.95,1.14863049153645)) ;
#20354=CARTESIAN_POINT('Origin',(-8.72471478008953,-0.8,1.14863049153645)) ;
#20355=CARTESIAN_POINT('Origin',(-8.72471478008953,-0.8,1.14863049153645)) ;
#20356=CARTESIAN_POINT('Origin',(-8.13013988609932,-0.95,3.36761420481279)) ;
#20357=CARTESIAN_POINT('',(-8.28013988609932,-1.,3.36761420481279)) ;
#20358=CARTESIAN_POINT('Origin',(-8.13013988609932,-1.,3.36761420481279)) ;
#20359=CARTESIAN_POINT('',(-8.28013988609932,-0.8,3.36761420481279)) ;
#20360=CARTESIAN_POINT('',(-8.28013988609932,-0.95,3.36761420481279)) ;
#20361=CARTESIAN_POINT('Origin',(-8.13013988609932,-0.8,3.36761420481279)) ;
#20362=CARTESIAN_POINT('Origin',(-8.13013988609932,-0.8,3.36761420481279)) ;
#20363=CARTESIAN_POINT('Origin',(-6.98150939456287,-0.95,5.35710057527674)) ;
#20364=CARTESIAN_POINT('',(-7.13150939456287,-1.,5.35710057527674)) ;
#20365=CARTESIAN_POINT('Origin',(-6.98150939456287,-1.,5.35710057527674)) ;
#20366=CARTESIAN_POINT('',(-7.13150939456287,-0.8,5.35710057527674)) ;
#20367=CARTESIAN_POINT('',(-7.13150939456287,-0.95,5.35710057527674)) ;
#20368=CARTESIAN_POINT('Origin',(-6.98150939456287,-0.8,5.35710057527674)) ;
#20369=CARTESIAN_POINT('Origin',(-6.98150939456287,-0.8,5.35710057527674)) ;
#20370=CARTESIAN_POINT('Origin',(-5.35710057527674,-0.95,6.98150939456287)) ;
#20371=CARTESIAN_POINT('',(-5.50710057527674,-1.,6.98150939456287)) ;
#20372=CARTESIAN_POINT('Origin',(-5.35710057527674,-1.,6.98150939456287)) ;
#20373=CARTESIAN_POINT('',(-5.50710057527674,-0.8,6.98150939456287)) ;
#20374=CARTESIAN_POINT('',(-5.50710057527674,-0.95,6.98150939456287)) ;
#20375=CARTESIAN_POINT('Origin',(-5.35710057527674,-0.8,6.98150939456287)) ;
#20376=CARTESIAN_POINT('Origin',(-5.35710057527674,-0.8,6.98150939456287)) ;
#20377=CARTESIAN_POINT('Origin',(-3.36761420481279,-0.95,8.13013988609932)) ;
#20378=CARTESIAN_POINT('',(-3.51761420481279,-1.,8.13013988609932)) ;
#20379=CARTESIAN_POINT('Origin',(-3.36761420481279,-1.,8.13013988609932)) ;
#20380=CARTESIAN_POINT('',(-3.51761420481279,-0.8,8.13013988609932)) ;
#20381=CARTESIAN_POINT('',(-3.51761420481279,-0.95,8.13013988609932)) ;
#20382=CARTESIAN_POINT('Origin',(-3.36761420481279,-0.8,8.13013988609932)) ;
#20383=CARTESIAN_POINT('Origin',(-3.36761420481279,-0.8,8.13013988609932)) ;
#20384=CARTESIAN_POINT('Origin',(-1.14863049153645,-0.95,8.72471478008953)) ;
#20385=CARTESIAN_POINT('',(-1.29863049153645,-1.,8.72471478008953)) ;
#20386=CARTESIAN_POINT('Origin',(-1.14863049153645,-1.,8.72471478008953)) ;
#20387=CARTESIAN_POINT('',(-1.29863049153645,-0.8,8.72471478008953)) ;
#20388=CARTESIAN_POINT('',(-1.29863049153645,-0.95,8.72471478008953)) ;
#20389=CARTESIAN_POINT('Origin',(-1.14863049153645,-0.8,8.72471478008953)) ;
#20390=CARTESIAN_POINT('Origin',(-1.14863049153645,-0.8,8.72471478008953)) ;
#20391=CARTESIAN_POINT('Origin',(1.14863049153646,-0.95,8.72471478008953)) ;
#20392=CARTESIAN_POINT('',(0.998630491536455,-1.,8.72471478008953)) ;
#20393=CARTESIAN_POINT('Origin',(1.14863049153646,-1.,8.72471478008953)) ;
#20394=CARTESIAN_POINT('',(0.998630491536455,-0.8,8.72471478008953)) ;
#20395=CARTESIAN_POINT('',(0.998630491536455,-0.95,8.72471478008953)) ;
#20396=CARTESIAN_POINT('Origin',(1.14863049153646,-0.8,8.72471478008953)) ;
#20397=CARTESIAN_POINT('Origin',(1.14863049153646,-0.8,8.72471478008953)) ;
#20398=CARTESIAN_POINT('Origin',(3.36761420481279,-0.95,8.13013988609932)) ;
#20399=CARTESIAN_POINT('',(3.21761420481279,-1.,8.13013988609932)) ;
#20400=CARTESIAN_POINT('Origin',(3.36761420481279,-1.,8.13013988609932)) ;
#20401=CARTESIAN_POINT('',(3.21761420481279,-0.8,8.13013988609932)) ;
#20402=CARTESIAN_POINT('',(3.21761420481279,-0.95,8.13013988609932)) ;
#20403=CARTESIAN_POINT('Origin',(3.36761420481279,-0.8,8.13013988609932)) ;
#20404=CARTESIAN_POINT('Origin',(3.36761420481279,-0.8,8.13013988609932)) ;
#20405=CARTESIAN_POINT('Origin',(5.35710057527674,-0.95,6.98150939456287)) ;
#20406=CARTESIAN_POINT('',(5.20710057527674,-1.,6.98150939456287)) ;
#20407=CARTESIAN_POINT('Origin',(5.35710057527674,-1.,6.98150939456287)) ;
#20408=CARTESIAN_POINT('',(5.20710057527674,-0.8,6.98150939456287)) ;
#20409=CARTESIAN_POINT('',(5.20710057527674,-0.95,6.98150939456287)) ;
#20410=CARTESIAN_POINT('Origin',(5.35710057527674,-0.8,6.98150939456287)) ;
#20411=CARTESIAN_POINT('Origin',(5.35710057527674,-0.8,6.98150939456287)) ;
#20412=CARTESIAN_POINT('Origin',(6.98150939456287,-0.95,5.35710057527674)) ;
#20413=CARTESIAN_POINT('',(6.83150939456287,-1.,5.35710057527674)) ;
#20414=CARTESIAN_POINT('Origin',(6.98150939456287,-1.,5.35710057527674)) ;
#20415=CARTESIAN_POINT('',(6.83150939456287,-0.8,5.35710057527674)) ;
#20416=CARTESIAN_POINT('',(6.83150939456287,-0.95,5.35710057527674)) ;
#20417=CARTESIAN_POINT('Origin',(6.98150939456287,-0.8,5.35710057527674)) ;
#20418=CARTESIAN_POINT('Origin',(6.98150939456287,-0.8,5.35710057527674)) ;
#20419=CARTESIAN_POINT('Origin',(8.13013988609932,-0.95,3.36761420481279)) ;
#20420=CARTESIAN_POINT('',(7.98013988609932,-1.,3.36761420481279)) ;
#20421=CARTESIAN_POINT('Origin',(8.13013988609932,-1.,3.36761420481279)) ;
#20422=CARTESIAN_POINT('',(7.98013988609932,-0.8,3.36761420481279)) ;
#20423=CARTESIAN_POINT('',(7.98013988609932,-0.95,3.36761420481279)) ;
#20424=CARTESIAN_POINT('Origin',(8.13013988609932,-0.8,3.36761420481279)) ;
#20425=CARTESIAN_POINT('Origin',(8.13013988609932,-0.8,3.36761420481279)) ;
#20426=CARTESIAN_POINT('Origin',(8.72471478008953,-0.95,1.14863049153645)) ;
#20427=CARTESIAN_POINT('',(8.57471478008953,-1.,1.14863049153645)) ;
#20428=CARTESIAN_POINT('Origin',(8.72471478008953,-1.,1.14863049153645)) ;
#20429=CARTESIAN_POINT('',(8.57471478008953,-0.8,1.14863049153645)) ;
#20430=CARTESIAN_POINT('',(8.57471478008953,-0.95,1.14863049153645)) ;
#20431=CARTESIAN_POINT('Origin',(8.72471478008953,-0.8,1.14863049153645)) ;
#20432=CARTESIAN_POINT('Origin',(8.72471478008953,-0.8,1.14863049153645)) ;
#20433=CARTESIAN_POINT('Origin',(8.5001472713438,-0.65,-2.27760759690218)) ;
#20434=CARTESIAN_POINT('',(8.1001472713438,-1.,-2.27760759690218)) ;
#20435=CARTESIAN_POINT('Origin',(8.5001472713438,-1.,-2.27760759690218)) ;
#20436=CARTESIAN_POINT('',(8.1001472713438,-0.3,-2.27760759690218)) ;
#20437=CARTESIAN_POINT('',(8.1001472713438,-0.65,-2.27760759690218)) ;
#20438=CARTESIAN_POINT('Origin',(8.5001472713438,-0.3,-2.27760759690218)) ;
#20439=CARTESIAN_POINT('Origin',(7.62102355330306,-0.65,-4.4)) ;
#20440=CARTESIAN_POINT('',(7.22102355330306,-1.,-4.4)) ;
#20441=CARTESIAN_POINT('Origin',(7.62102355330306,-1.,-4.4)) ;
#20442=CARTESIAN_POINT('',(7.22102355330306,-0.3,-4.4)) ;
#20443=CARTESIAN_POINT('',(7.22102355330306,-0.65,-4.4)) ;
#20444=CARTESIAN_POINT('Origin',(7.62102355330306,-0.3,-4.4)) ;
#20445=CARTESIAN_POINT('Origin',(6.22253967444162,-0.65,-6.22253967444162)) ;
#20446=CARTESIAN_POINT('',(5.82253967444162,-1.,-6.22253967444162)) ;
#20447=CARTESIAN_POINT('Origin',(6.22253967444162,-1.,-6.22253967444162)) ;
#20448=CARTESIAN_POINT('',(5.82253967444162,-0.3,-6.22253967444162)) ;
#20449=CARTESIAN_POINT('',(5.82253967444162,-0.65,-6.22253967444162)) ;
#20450=CARTESIAN_POINT('Origin',(6.22253967444162,-0.3,-6.22253967444162)) ;
#20451=CARTESIAN_POINT('Origin',(4.4,-0.65,-7.62102355330306)) ;
#20452=CARTESIAN_POINT('',(4.,-1.,-7.62102355330306)) ;
#20453=CARTESIAN_POINT('Origin',(4.4,-1.,-7.62102355330306)) ;
#20454=CARTESIAN_POINT('',(4.,-0.3,-7.62102355330306)) ;
#20455=CARTESIAN_POINT('',(4.,-0.65,-7.62102355330306)) ;
#20456=CARTESIAN_POINT('Origin',(4.4,-0.3,-7.62102355330306)) ;
#20457=CARTESIAN_POINT('Origin',(2.27760759690218,-0.65,-8.5001472713438)) ;
#20458=CARTESIAN_POINT('',(1.87760759690218,-1.,-8.5001472713438)) ;
#20459=CARTESIAN_POINT('Origin',(2.27760759690218,-1.,-8.5001472713438)) ;
#20460=CARTESIAN_POINT('',(1.87760759690218,-0.3,-8.5001472713438)) ;
#20461=CARTESIAN_POINT('',(1.87760759690218,-0.65,-8.5001472713438)) ;
#20462=CARTESIAN_POINT('Origin',(2.27760759690218,-0.3,-8.5001472713438)) ;
#20463=CARTESIAN_POINT('Origin',(-1.61653377487451E-15,-0.65,-8.8)) ;
#20464=CARTESIAN_POINT('',(-0.400000000000002,-1.,-8.8)) ;
#20465=CARTESIAN_POINT('Origin',(-1.61653377487451E-15,-1.,-8.8)) ;
#20466=CARTESIAN_POINT('',(-0.400000000000002,-0.3,-8.8)) ;
#20467=CARTESIAN_POINT('',(-0.400000000000002,-0.65,-8.8)) ;
#20468=CARTESIAN_POINT('Origin',(-1.61653377487451E-15,-0.3,-8.8)) ;
#20469=CARTESIAN_POINT('Origin',(-2.27760759690218,-0.65,-8.5001472713438)) ;
#20470=CARTESIAN_POINT('',(-2.67760759690218,-1.,-8.5001472713438)) ;
#20471=CARTESIAN_POINT('Origin',(-2.27760759690218,-1.,-8.5001472713438)) ;
#20472=CARTESIAN_POINT('',(-2.67760759690218,-0.3,-8.5001472713438)) ;
#20473=CARTESIAN_POINT('',(-2.67760759690218,-0.65,-8.5001472713438)) ;
#20474=CARTESIAN_POINT('Origin',(-2.27760759690218,-0.3,-8.5001472713438)) ;
#20475=CARTESIAN_POINT('Origin',(-4.4,-0.65,-7.62102355330306)) ;
#20476=CARTESIAN_POINT('',(-4.80000000000001,-1.,-7.62102355330306)) ;
#20477=CARTESIAN_POINT('Origin',(-4.4,-1.,-7.62102355330306)) ;
#20478=CARTESIAN_POINT('',(-4.80000000000001,-0.3,-7.62102355330306)) ;
#20479=CARTESIAN_POINT('',(-4.80000000000001,-0.65,-7.62102355330306)) ;
#20480=CARTESIAN_POINT('Origin',(-4.4,-0.3,-7.62102355330306)) ;
#20481=CARTESIAN_POINT('Origin',(-6.22253967444162,-0.65,-6.22253967444162)) ;
#20482=CARTESIAN_POINT('',(-6.62253967444162,-1.,-6.22253967444162)) ;
#20483=CARTESIAN_POINT('Origin',(-6.22253967444162,-1.,-6.22253967444162)) ;
#20484=CARTESIAN_POINT('',(-6.62253967444162,-0.3,-6.22253967444162)) ;
#20485=CARTESIAN_POINT('',(-6.62253967444162,-0.65,-6.22253967444162)) ;
#20486=CARTESIAN_POINT('Origin',(-6.22253967444162,-0.3,-6.22253967444162)) ;
#20487=CARTESIAN_POINT('Origin',(-7.62102355330306,-0.65,-4.4)) ;
#20488=CARTESIAN_POINT('',(-8.02102355330306,-1.,-4.4)) ;
#20489=CARTESIAN_POINT('Origin',(-7.62102355330306,-1.,-4.4)) ;
#20490=CARTESIAN_POINT('',(-8.02102355330306,-0.3,-4.4)) ;
#20491=CARTESIAN_POINT('',(-8.02102355330306,-0.65,-4.4)) ;
#20492=CARTESIAN_POINT('Origin',(-7.62102355330306,-0.3,-4.4)) ;
#20493=CARTESIAN_POINT('Origin',(-8.5001472713438,-0.65,-2.27760759690218)) ;
#20494=CARTESIAN_POINT('',(-8.9001472713438,-1.,-2.27760759690218)) ;
#20495=CARTESIAN_POINT('Origin',(-8.5001472713438,-1.,-2.27760759690218)) ;
#20496=CARTESIAN_POINT('',(-8.9001472713438,-0.3,-2.27760759690218)) ;
#20497=CARTESIAN_POINT('',(-8.9001472713438,-0.65,-2.27760759690218)) ;
#20498=CARTESIAN_POINT('Origin',(-8.5001472713438,-0.3,-2.27760759690218)) ;
#20499=CARTESIAN_POINT('Origin',(-8.8,-0.65,1.07768918324967E-15)) ;
#20500=CARTESIAN_POINT('',(-9.2,-1.,1.12667505521557E-15)) ;
#20501=CARTESIAN_POINT('Origin',(-8.8,-1.,1.07768918324967E-15)) ;
#20502=CARTESIAN_POINT('',(-9.2,-0.3,1.02870331128378E-15)) ;
#20503=CARTESIAN_POINT('',(-9.2,-0.65,1.12667505521557E-15)) ;
#20504=CARTESIAN_POINT('Origin',(-8.8,-0.3,1.07768918324967E-15)) ;
#20505=CARTESIAN_POINT('Origin',(-8.5001472713438,-0.65,2.27760759690219)) ;
#20506=CARTESIAN_POINT('',(-8.9001472713438,-1.,2.27760759690219)) ;
#20507=CARTESIAN_POINT('Origin',(-8.5001472713438,-1.,2.27760759690219)) ;
#20508=CARTESIAN_POINT('',(-8.9001472713438,-0.3,2.27760759690219)) ;
#20509=CARTESIAN_POINT('',(-8.9001472713438,-0.65,2.27760759690219)) ;
#20510=CARTESIAN_POINT('Origin',(-8.5001472713438,-0.3,2.27760759690219)) ;
#20511=CARTESIAN_POINT('Origin',(-7.62102355330306,-0.65,4.4)) ;
#20512=CARTESIAN_POINT('',(-8.02102355330306,-1.,4.4)) ;
#20513=CARTESIAN_POINT('Origin',(-7.62102355330306,-1.,4.4)) ;
#20514=CARTESIAN_POINT('',(-8.02102355330306,-0.3,4.4)) ;
#20515=CARTESIAN_POINT('',(-8.02102355330306,-0.65,4.4)) ;
#20516=CARTESIAN_POINT('Origin',(-7.62102355330306,-0.3,4.4)) ;
#20517=CARTESIAN_POINT('Origin',(-6.22253967444162,-0.65,6.22253967444162)) ;
#20518=CARTESIAN_POINT('',(-6.62253967444162,-1.,6.22253967444162)) ;
#20519=CARTESIAN_POINT('Origin',(-6.22253967444162,-1.,6.22253967444162)) ;
#20520=CARTESIAN_POINT('',(-6.62253967444162,-0.3,6.22253967444162)) ;
#20521=CARTESIAN_POINT('',(-6.62253967444162,-0.65,6.22253967444162)) ;
#20522=CARTESIAN_POINT('Origin',(-6.22253967444162,-0.3,6.22253967444162)) ;
#20523=CARTESIAN_POINT('Origin',(-4.4,-0.65,7.62102355330306)) ;
#20524=CARTESIAN_POINT('',(-4.8,-1.,7.62102355330306)) ;
#20525=CARTESIAN_POINT('Origin',(-4.4,-1.,7.62102355330306)) ;
#20526=CARTESIAN_POINT('',(-4.8,-0.3,7.62102355330306)) ;
#20527=CARTESIAN_POINT('',(-4.8,-0.65,7.62102355330306)) ;
#20528=CARTESIAN_POINT('Origin',(-4.4,-0.3,7.62102355330306)) ;
#20529=CARTESIAN_POINT('Origin',(-2.27760759690218,-0.65,8.5001472713438)) ;
#20530=CARTESIAN_POINT('',(-2.67760759690218,-1.,8.5001472713438)) ;
#20531=CARTESIAN_POINT('Origin',(-2.27760759690218,-1.,8.5001472713438)) ;
#20532=CARTESIAN_POINT('',(-2.67760759690218,-0.3,8.5001472713438)) ;
#20533=CARTESIAN_POINT('',(-2.67760759690218,-0.65,8.5001472713438)) ;
#20534=CARTESIAN_POINT('Origin',(-2.27760759690218,-0.3,8.5001472713438)) ;
#20535=CARTESIAN_POINT('Origin',(5.38844591624835E-16,-0.65,8.8)) ;
#20536=CARTESIAN_POINT('',(-0.399999999999999,-1.,8.8)) ;
#20537=CARTESIAN_POINT('Origin',(5.38844591624835E-16,-1.,8.8)) ;
#20538=CARTESIAN_POINT('',(-0.399999999999999,-0.3,8.8)) ;
#20539=CARTESIAN_POINT('',(-0.399999999999999,-0.65,8.8)) ;
#20540=CARTESIAN_POINT('Origin',(5.38844591624835E-16,-0.3,8.8)) ;
#20541=CARTESIAN_POINT('Origin',(2.27760759690218,-0.65,8.5001472713438)) ;
#20542=CARTESIAN_POINT('',(1.87760759690218,-1.,8.5001472713438)) ;
#20543=CARTESIAN_POINT('Origin',(2.27760759690218,-1.,8.5001472713438)) ;
#20544=CARTESIAN_POINT('',(1.87760759690218,-0.3,8.5001472713438)) ;
#20545=CARTESIAN_POINT('',(1.87760759690218,-0.65,8.5001472713438)) ;
#20546=CARTESIAN_POINT('Origin',(2.27760759690218,-0.3,8.5001472713438)) ;
#20547=CARTESIAN_POINT('Origin',(4.4,-0.65,7.62102355330306)) ;
#20548=CARTESIAN_POINT('',(4.,-1.,7.62102355330306)) ;
#20549=CARTESIAN_POINT('Origin',(4.4,-1.,7.62102355330306)) ;
#20550=CARTESIAN_POINT('',(4.,-0.3,7.62102355330306)) ;
#20551=CARTESIAN_POINT('',(4.,-0.65,7.62102355330306)) ;
#20552=CARTESIAN_POINT('Origin',(4.4,-0.3,7.62102355330306)) ;
#20553=CARTESIAN_POINT('Origin',(6.22253967444162,-0.65,6.22253967444162)) ;
#20554=CARTESIAN_POINT('',(5.82253967444162,-1.,6.22253967444162)) ;
#20555=CARTESIAN_POINT('Origin',(6.22253967444162,-1.,6.22253967444162)) ;
#20556=CARTESIAN_POINT('',(5.82253967444162,-0.3,6.22253967444162)) ;
#20557=CARTESIAN_POINT('',(5.82253967444162,-0.65,6.22253967444162)) ;
#20558=CARTESIAN_POINT('Origin',(6.22253967444162,-0.3,6.22253967444162)) ;
#20559=CARTESIAN_POINT('Origin',(7.62102355330306,-0.65,4.4)) ;
#20560=CARTESIAN_POINT('',(7.22102355330306,-1.,4.4)) ;
#20561=CARTESIAN_POINT('Origin',(7.62102355330306,-1.,4.4)) ;
#20562=CARTESIAN_POINT('',(7.22102355330306,-0.3,4.4)) ;
#20563=CARTESIAN_POINT('',(7.22102355330306,-0.65,4.4)) ;
#20564=CARTESIAN_POINT('Origin',(7.62102355330306,-0.3,4.4)) ;
#20565=CARTESIAN_POINT('Origin',(8.5001472713438,-0.65,2.27760759690218)) ;
#20566=CARTESIAN_POINT('',(8.1001472713438,-1.,2.27760759690218)) ;
#20567=CARTESIAN_POINT('Origin',(8.5001472713438,-1.,2.27760759690218)) ;
#20568=CARTESIAN_POINT('',(8.1001472713438,-0.3,2.27760759690218)) ;
#20569=CARTESIAN_POINT('',(8.1001472713438,-0.65,2.27760759690218)) ;
#20570=CARTESIAN_POINT('Origin',(8.5001472713438,-0.3,2.27760759690218)) ;
#20571=CARTESIAN_POINT('Origin',(8.8,-0.65,0.)) ;
#20572=CARTESIAN_POINT('',(8.4,-1.,4.89858719658941E-17)) ;
#20573=CARTESIAN_POINT('Origin',(8.8,-1.,0.)) ;
#20574=CARTESIAN_POINT('',(8.4,-0.3,-4.89858719658941E-17)) ;
#20575=CARTESIAN_POINT('',(8.4,-0.65,4.89858719658941E-17)) ;
#20576=CARTESIAN_POINT('Origin',(8.8,-0.3,0.)) ;
#20577=CARTESIAN_POINT('Origin',(1.55884572681199,-0.65,-0.900000000000001)) ;
#20578=CARTESIAN_POINT('',(1.34384572681199,-1.,-0.900000000000001)) ;
#20579=CARTESIAN_POINT('Origin',(1.55884572681199,-1.,-0.900000000000001)) ;
#20580=CARTESIAN_POINT('',(1.34384572681199,-0.3,-0.900000000000001)) ;
#20581=CARTESIAN_POINT('',(1.34384572681199,-0.65,-0.900000000000001)) ;
#20582=CARTESIAN_POINT('Origin',(1.55884572681199,-0.3,-0.900000000000001)) ;
#20583=CARTESIAN_POINT('Origin',(-1.55884572681199,-0.65,-0.9)) ;
#20584=CARTESIAN_POINT('',(-1.77384572681199,-1.,-0.9)) ;
#20585=CARTESIAN_POINT('Origin',(-1.55884572681199,-1.,-0.9)) ;
#20586=CARTESIAN_POINT('',(-1.77384572681199,-0.3,-0.9)) ;
#20587=CARTESIAN_POINT('',(-1.77384572681199,-0.65,-0.9)) ;
#20588=CARTESIAN_POINT('Origin',(-1.55884572681199,-0.3,-0.9)) ;
#20589=CARTESIAN_POINT('Origin',(1.10218211923262E-16,-0.65,1.8)) ;
#20590=CARTESIAN_POINT('',(-0.215,-1.,1.8)) ;
#20591=CARTESIAN_POINT('Origin',(1.10218211923262E-16,-1.,1.8)) ;
#20592=CARTESIAN_POINT('',(-0.215,-0.3,1.8)) ;
#20593=CARTESIAN_POINT('',(-0.215,-0.65,1.8)) ;
#20594=CARTESIAN_POINT('Origin',(1.10218211923262E-16,-0.3,1.8)) ;
#20595=CARTESIAN_POINT('Origin',(0.,-0.65,0.)) ;
#20596=CARTESIAN_POINT('',(-0.51,-1.,6.2456986756515E-17)) ;
#20597=CARTESIAN_POINT('Origin',(0.,-1.,0.)) ;
#20598=CARTESIAN_POINT('',(-0.51,-0.3,-6.2456986756515E-17)) ;
#20599=CARTESIAN_POINT('',(-0.51,-0.65,6.2456986756515E-17)) ;
#20600=CARTESIAN_POINT('Origin',(0.,-0.3,0.)) ;
#20601=CARTESIAN_POINT('Origin',(0.,-0.65,0.)) ;
#20602=CARTESIAN_POINT('',(-10.,-0.3,1.22464679914735E-15)) ;
#20603=CARTESIAN_POINT('Origin',(0.,-0.3,0.)) ;
#20604=CARTESIAN_POINT('',(-10.,-1.,1.22464679914735E-15)) ;
#20605=CARTESIAN_POINT('',(-10.,-0.65,1.22464679914735E-15)) ;
#20606=CARTESIAN_POINT('Origin',(0.,-1.,0.)) ;
#20607=CARTESIAN_POINT('Origin',(0.,-1.,0.)) ;
#20608=CARTESIAN_POINT('Origin',(0.,-0.3,0.)) ;
#24540=UNCERTAINTY_MEASURE_WITH_UNIT(LENGTH_MEASURE(0.001),#24629,
'DISTANCE_ACCURACY_VALUE',
'Maximum model space distance between geometric entities at asserted c
onnectivities') ;
#24580=UNCERTAINTY_MEASURE_WITH_UNIT(LENGTH_MEASURE(0.001),#24629,
'DISTANCE_ACCURACY_VALUE',
'Maximum model space distance between geometric entities at asserted c
onnectivities') ;
#24588=(
GEOMETRIC_REPRESENTATION_CONTEXT(3)
GLOBAL_UNCERTAINTY_ASSIGNED_CONTEXT((#24540))
GLOBAL_UNIT_ASSIGNED_CONTEXT((#24629,#24631,#24632))
REPRESENTATION_CONTEXT('','3D')
) ;
#24628=(
GEOMETRIC_REPRESENTATION_CONTEXT(3)
GLOBAL_UNCERTAINTY_ASSIGNED_CONTEXT((#24580))
GLOBAL_UNIT_ASSIGNED_CONTEXT((#24629,#24631,#24632))
REPRESENTATION_CONTEXT('','3D')
) ;
#24629=(
LENGTH_UNIT()
NAMED_UNIT(*)
SI_UNIT(.CENTI.,.METRE.)
) ;
#24631=(
NAMED_UNIT(*)
PLANE_ANGLE_UNIT()
SI_UNIT($,.RADIAN.)
) ;
#24632=(
NAMED_UNIT(*)
SI_UNIT($,.STERADIAN.)
SOLID_ANGLE_UNIT()
) ;
#24640=SHAPE_DEFINITION_REPRESENTATION(#24687,#24798) ;
#24687=PRODUCT_DEFINITION_SHAPE('',$,#24846) ;
#24798=SHAPE_REPRESENTATION('',(#13875),#24588) ;
#24838=PRODUCT_DEFINITION_CONTEXT('part definition',#24981,'design') ;
#24846=PRODUCT_DEFINITION('ROTATING_SEEDING_PLATE',
'ROTATING_SEEDING_PLATE',#24893,#24838) ;
#24893=PRODUCT_DEFINITION_FORMATION('',$,#24990) ;
#24981=APPLICATION_CONTEXT(
'Core Data for Automotive Mechanical Design Process') ;
#24982=PRODUCT_CONTEXT('part definition',#24981,'mechanical') ;
#24990=PRODUCT('ROTATING_SEEDING_PLATE','ROTATING_SEEDING_PLATE',$,(#24982)) ;
#25034=PRESENTATION_STYLE_ASSIGNMENT((#25044)) ;
#25044=SURFACE_STYLE_USAGE(.BOTH.,#25054) ;
#25054=SURFACE_SIDE_STYLE('',(#25064)) ;
#25064=SURFACE_STYLE_FILL_AREA(#25074) ;
#25074=FILL_AREA_STYLE('Stainless Steel - Satin',(#25084)) ;
#25084=FILL_AREA_STYLE_COLOUR('Stainless Steel - Satin',#25094) ;
#25094=COLOUR_RGB('Stainless Steel - Satin', 0.31764706, 0.68627451, 0.89019608) ;
ENDSEC;
END-ISO-10303-21;
